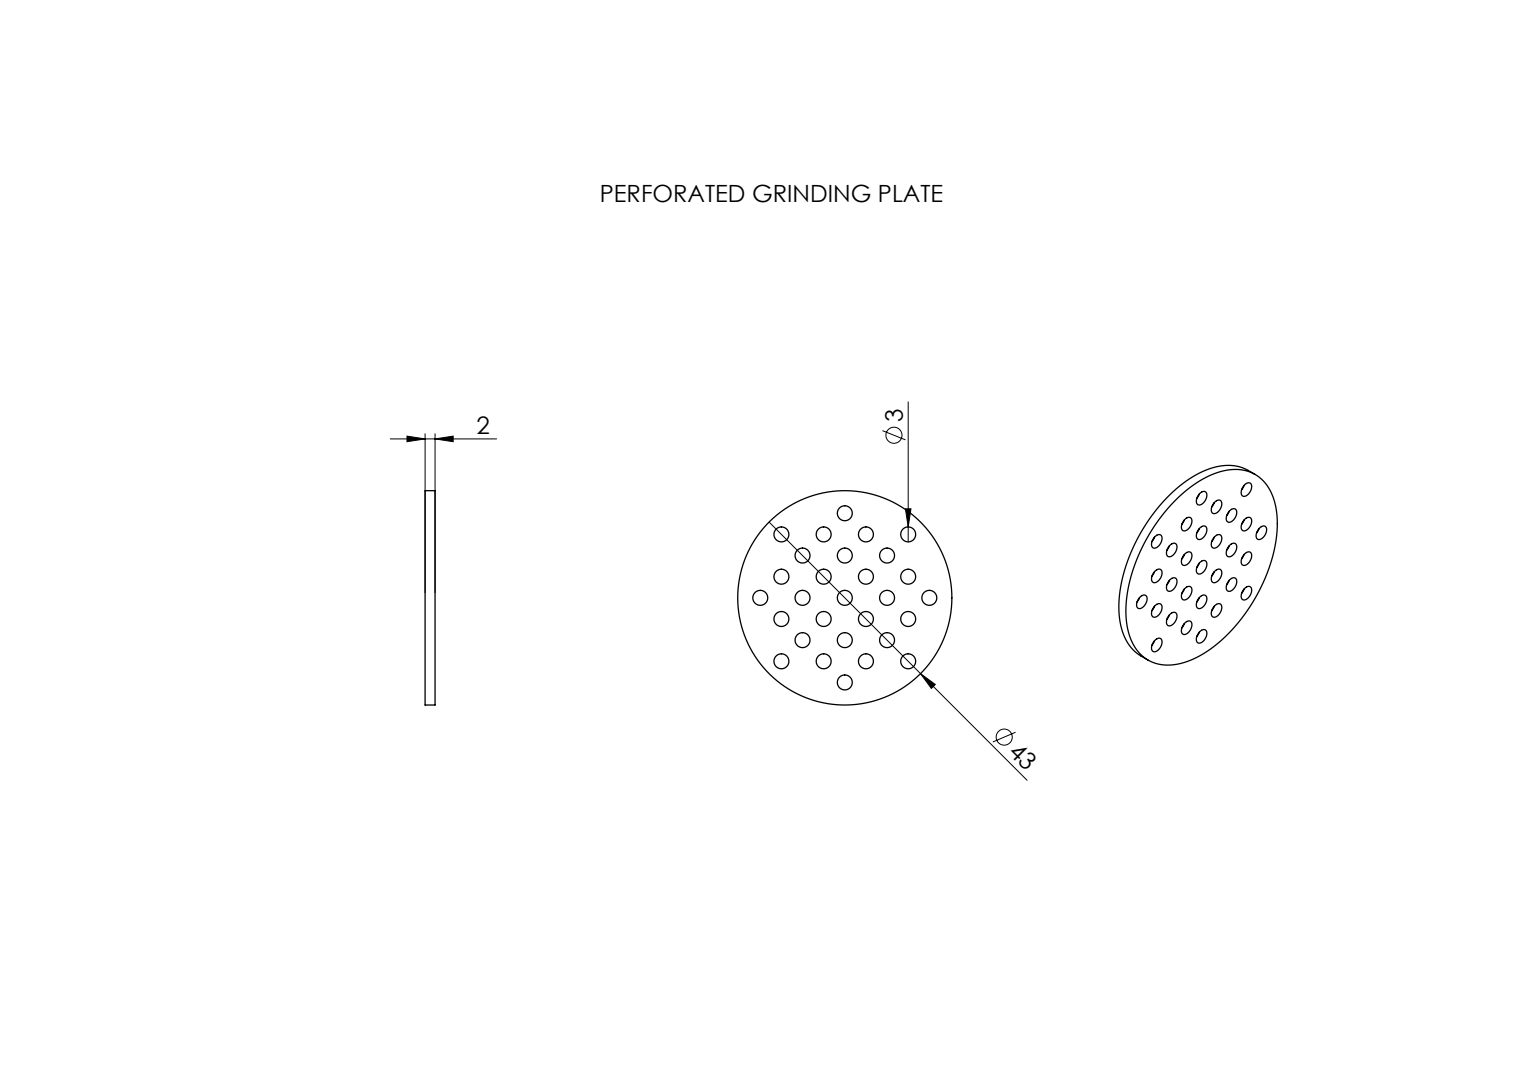
ISO-10303-21;
HEADER;
FILE_DESCRIPTION (('STEP AP214'),
    '1' );
FILE_NAME ('perforated grinding plate.step',
    '2026-10-22T10:02:39',
    ( '' ),
    ( '' ),
    'SwSTEP 2.0',
    'SolidWorks 2026',
    '' );
FILE_SCHEMA (( 'AUTOMOTIVE_DESIGN' ));
ENDSEC;

DATA;
#7=CIRCLE ( 'NONE', #1554, 1.500000000000001332 ) ;
#9=ORIENTED_EDGE ( 'NONE', *, *, #6036, .T. ) ;
#14=AXIS2_PLACEMENT_3D ( 'NONE', #9720, #5068, #10559 ) ;
#19=VERTEX_POINT ( 'NONE', #7735 ) ;
#21=CARTESIAN_POINT ( 'NONE',  ( -78.00000000000001421, 59.24264068711927678, 4.242644059037073312 ) ) ;
#27=DIRECTION ( 'NONE',  ( 0.000000000000000000, 0.000000000000000000, 1.000000000000000000 ) ) ;
#28=CARTESIAN_POINT ( 'NONE',  ( -78.00000000000001421, 50.75735931288069480, -11.22791868944003824 ) ) ;
#29=DIRECTION ( 'NONE',  ( -1.000000000000000000, -0.000000000000000000, -0.000000000000000000 ) ) ;
#34=CARTESIAN_POINT ( 'NONE',  ( -80.00000000000001421, 63.48528137423857487, 8.485284746156350977 ) ) ;
#36=DIRECTION ( 'NONE',  ( 0.000000000000000000, 1.000000000000000000, 0.000000000000000000 ) ) ;
#43=VERTEX_POINT ( 'NONE', #10470 ) ;
#61=ADVANCED_FACE ( 'NONE', ( #1382, #293, #5043, #8690, #5765, #7618, #472, #11246, #4861, #6728, #10360, #351, #7675, #5881, #9524, #9811, #11776, #5272, #7139, #8090, #4373, #7912, #9698, #7079, #1495, #5216, #7192, #9040, #7965, #8982 ), #11541, .F. ) ;
#68=FACE_OUTER_BOUND ( 'NONE', #814, .T. ) ;
#69=VERTEX_POINT ( 'NONE', #11601 ) ;
#72=EDGE_CURVE ( 'NONE', #8769, #5516, #701, .T. ) ;
#79=EDGE_LOOP ( 'NONE', ( #6944, #10404, #6581, #2124 ) ) ;
#88=LINE ( 'NONE', #7135, #10139 ) ;
#89=VERTEX_POINT ( 'NONE', #9752 ) ;
#90=CARTESIAN_POINT ( 'NONE',  ( -78.00000000000002842, 54.99999999999998579, 15.47056612039490986 ) ) ;
#96=VERTEX_POINT ( 'NONE', #6118 ) ;
#102=CARTESIAN_POINT ( 'NONE',  ( -80.00000000000002842, 38.02943725152282184, 3.371917797929946392E-06 ) ) ;
#114=ORIENTED_EDGE ( 'NONE', *, *, #10655, .T. ) ;
#118=CIRCLE ( 'NONE', #8173, 1.500000000000001332 ) ;
#119=CARTESIAN_POINT ( 'NONE',  ( -78.00000000000001421, 50.75735931288069480, -12.72791868944003824 ) ) ;
#128=ORIENTED_EDGE ( 'NONE', *, *, #8290, .T. ) ;
#130=CYLINDRICAL_SURFACE ( 'NONE', #5375, 1.500000000000000000 ) ;
#150=CYLINDRICAL_SURFACE ( 'NONE', #7865, 1.499999999999999556 ) ;
#152=ORIENTED_EDGE ( 'NONE', *, *, #4340, .T. ) ;
#169=CIRCLE ( 'NONE', #3240, 1.500000000000001332 ) ;
#172=AXIS2_PLACEMENT_3D ( 'NONE', #8865, #9866, #7078 ) ;
#183=CYLINDRICAL_SURFACE ( 'NONE', #11845, 1.500000000000000444 ) ;
#195=VECTOR ( 'NONE', #5572, 1000.000000000000000 ) ;
#202=PRESENTATION_STYLE_ASSIGNMENT (( #2843 ) ) ;
#206=EDGE_CURVE ( 'NONE', #6519, #11654, #6983, .T. ) ;
#232=ORIENTED_EDGE ( 'NONE', *, *, #8402, .T. ) ;
#241=VERTEX_POINT ( 'NONE', #2085 ) ;
#244=LINE ( 'NONE', #4871, #4047 ) ;
#245=FACE_BOUND ( 'NONE', #9079, .T. ) ;
#247=DIRECTION ( 'NONE',  ( -1.000000000000000000, -0.000000000000000000, -0.000000000000000000 ) ) ;
#248=DIRECTION ( 'NONE',  ( -1.000000000000000000, -0.000000000000000000, -0.000000000000000000 ) ) ;
#250=CARTESIAN_POINT ( 'NONE',  ( -78.00000000000002842, 42.27207793864211283, -4.242637315201479353 ) ) ;
#252=ORIENTED_EDGE ( 'NONE', *, *, #5075, .F. ) ;
#255=DIRECTION ( 'NONE',  ( -1.000000000000000000, -0.000000000000000000, -0.000000000000000000 ) ) ;
#258=DIRECTION ( 'NONE',  ( 0.000000000000000000, 1.000000000000000000, 0.000000000000000000 ) ) ;
#263=ADVANCED_FACE ( 'NONE', ( #10291 ), #10352, .F. ) ;
#269=CYLINDRICAL_SURFACE ( 'NONE', #2101, 1.499999999999999556 ) ;
#282=DIRECTION ( 'NONE',  ( -1.000000000000000000, -0.000000000000000000, -0.000000000000000000 ) ) ;
#293=FACE_BOUND ( 'NONE', #10060, .T. ) ;
#299=EDGE_CURVE ( 'NONE', #11481, #8007, #11177, .T. ) ;
#302=AXIS2_PLACEMENT_3D ( 'NONE', #9626, #1421, #6826 ) ;
#314=CIRCLE ( 'NONE', #4535, 1.500000000000001332 ) ;
#320=CIRCLE ( 'NONE', #10069, 1.500000000000001332 ) ;
#322=VERTEX_POINT ( 'NONE', #10463 ) ;
#326=EDGE_LOOP ( 'NONE', ( #6442, #4542, #10386, #11390 ) ) ;
#330=CARTESIAN_POINT ( 'NONE',  ( -78.00000000000002842, 42.27207793864211283, -5.742637315201479353 ) ) ;
#332=DIRECTION ( 'NONE',  ( 0.000000000000000000, 0.000000000000000000, 1.000000000000000000 ) ) ;
#334=EDGE_LOOP ( 'NONE', ( #4076, #9464, #9647, #1105 ) ) ;
#341=ORIENTED_EDGE ( 'NONE', *, *, #3274, .F. ) ;
#345=CARTESIAN_POINT ( 'NONE',  ( -78.00000000000001421, 50.75735931288069480, -4.242637315201482906 ) ) ;
#348=EDGE_LOOP ( 'NONE', ( #11086, #2027, #10257, #10094 ) ) ;
#351=FACE_BOUND ( 'NONE', #8937, .T. ) ;
#356=CARTESIAN_POINT ( 'NONE',  ( -80.00000000000002842, 42.27207793864211283, -2.742637315201478909 ) ) ;
#362=AXIS2_PLACEMENT_3D ( 'NONE', #7929, #10661, #6136 ) ;
#369=CARTESIAN_POINT ( 'NONE',  ( -78.00000000000001421, 59.24264068711928388, -12.72791868944003824 ) ) ;
#382=EDGE_CURVE ( 'NONE', #9787, #911, #6720, .T. ) ;
#392=CYLINDRICAL_SURFACE ( 'NONE', #7755, 1.499999999999999556 ) ;
#395=CARTESIAN_POINT ( 'NONE',  ( -78.00000000000002842, 42.27207793864211283, 5.742644059037075088 ) ) ;
#404=ORIENTED_EDGE ( 'NONE', *, *, #2192, .T. ) ;
#411=ORIENTED_EDGE ( 'NONE', *, *, #7065, .F. ) ;
#424=CARTESIAN_POINT ( 'NONE',  ( -78.00000000000001421, 59.24264068711927678, -4.242637315201482906 ) ) ;
#430=VERTEX_POINT ( 'NONE', #4072 ) ;
#441=CARTESIAN_POINT ( 'NONE',  ( -78.00000000000001421, 59.24264068711927678, -4.242637315201482906 ) ) ;
#442=CARTESIAN_POINT ( 'NONE',  ( -78.00000000000001421, 59.24264068711927678, 5.742644059037073312 ) ) ;
#447=EDGE_CURVE ( 'NONE', #3965, #2443, #10013, .T. ) ;
#452=DIRECTION ( 'NONE',  ( -1.000000000000000000, -0.000000000000000000, -0.000000000000000000 ) ) ;
#460=CARTESIAN_POINT ( 'NONE',  ( -78.00000000000000000, 54.99999999999999289, 1.500003371917797201 ) ) ;
#469=ORIENTED_EDGE ( 'NONE', *, *, #6959, .T. ) ;
#471=FACE_OUTER_BOUND ( 'NONE', #3888, .T. ) ;
#472=FACE_BOUND ( 'NONE', #918, .T. ) ;
#479=EDGE_LOOP ( 'NONE', ( #6589, #1548 ) ) ;
#484=ORIENTED_EDGE ( 'NONE', *, *, #797, .F. ) ;
#490=AXIS2_PLACEMENT_3D ( 'NONE', #6892, #11533, #10461 ) ;
#491=EDGE_LOOP ( 'NONE', ( #6034, #9162, #10252, #4142 ) ) ;
#506=AXIS2_PLACEMENT_3D ( 'NONE', #833, #7216, #2766 ) ;
#512=ADVANCED_FACE ( 'NONE', ( #9745 ), #11473, .F. ) ;
#513=CYLINDRICAL_SURFACE ( 'NONE', #1318, 1.499999999999999556 ) ;
#517=AXIS2_PLACEMENT_3D ( 'NONE', #9788, #1581, #2488 ) ;
#518=VERTEX_POINT ( 'NONE', #5210 ) ;
#528=FACE_BOUND ( 'NONE', #6654, .T. ) ;
#537=DIRECTION ( 'NONE',  ( -1.000000000000000000, -0.000000000000000000, -0.000000000000000000 ) ) ;
#540=CYLINDRICAL_SURFACE ( 'NONE', #2889, 1.499999999999999556 ) ;
#548=DIRECTION ( 'NONE',  ( -1.000000000000000000, -0.000000000000000000, -0.000000000000000000 ) ) ;
#554=AXIS2_PLACEMENT_3D ( 'NONE', #4747, #2103, #5776 ) ;
#560=DIRECTION ( 'NONE',  ( -1.000000000000000000, -0.000000000000000000, -0.000000000000000000 ) ) ;
#571=ORIENTED_EDGE ( 'NONE', *, *, #3449, .F. ) ;
#572=AXIS2_PLACEMENT_3D ( 'NONE', #3732, #4757, #2835 ) ;
#575=ORIENTED_EDGE ( 'NONE', *, *, #6777, .T. ) ;
#581=DIRECTION ( 'NONE',  ( -1.000000000000000000, -0.000000000000000000, -0.000000000000000000 ) ) ;
#583=EDGE_LOOP ( 'NONE', ( #10142, #10451 ) ) ;
#587=EDGE_CURVE ( 'NONE', #96, #430, #9252, .T. ) ;
#590=VECTOR ( 'NONE', #3641, 1000.000000000000000 ) ;
#591=ORIENTED_EDGE ( 'NONE', *, *, #3891, .F. ) ;
#600=CYLINDRICAL_SURFACE ( 'NONE', #4784, 1.499999999999999556 ) ;
#615=DIRECTION ( 'NONE',  ( -1.000000000000000000, -0.000000000000000000, -0.000000000000000000 ) ) ;
#622=ORIENTED_EDGE ( 'NONE', *, *, #9614, .F. ) ;
#626=ORIENTED_EDGE ( 'NONE', *, *, #8896, .F. ) ;
#631=ORIENTED_EDGE ( 'NONE', *, *, #4619, .T. ) ;
#635=EDGE_LOOP ( 'NONE', ( #794, #9910 ) ) ;
#640=CARTESIAN_POINT ( 'NONE',  ( -78.00000000000002842, 46.51471862576140381, 1.500003371917798756 ) ) ;
#642=VERTEX_POINT ( 'NONE', #2683 ) ;
#650=CARTESIAN_POINT ( 'NONE',  ( -78.00000000000000000, 54.99999999999999289, 3.371917797062584654E-06 ) ) ;
#656=VERTEX_POINT ( 'NONE', #1719 ) ;
#660=ADVANCED_FACE ( 'NONE', ( #2854 ), #866, .F. ) ;
#666=ORIENTED_EDGE ( 'NONE', *, *, #2138, .F. ) ;
#669=CARTESIAN_POINT ( 'NONE',  ( -78.00000000000001421, 63.48528137423857487, 3.371917795327861178E-06 ) ) ;
#676=FACE_OUTER_BOUND ( 'NONE', #7285, .T. ) ;
#687=AXIS2_PLACEMENT_3D ( 'NONE', #9704, #7974, #8697 ) ;
#688=CARTESIAN_POINT ( 'NONE',  ( -78.00000000000001421, 71.97056274847716395, 3.371917795327861178E-06 ) ) ;
#700=DIRECTION ( 'NONE',  ( -1.000000000000000000, -0.000000000000000000, -0.000000000000000000 ) ) ;
#701=LINE ( 'NONE', #8025, #1937 ) ;
#704=ORIENTED_EDGE ( 'NONE', *, *, #10995, .F. ) ;
#709=DIRECTION ( 'NONE',  ( -1.000000000000000000, -0.000000000000000000, -0.000000000000000000 ) ) ;
#715=EDGE_LOOP ( 'NONE', ( #11097, #2302, #10666, #3336 ) ) ;
#721=DIRECTION ( 'NONE',  ( -1.000000000000000000, -0.000000000000000000, -0.000000000000000000 ) ) ;
#723=VERTEX_POINT ( 'NONE', #1773 ) ;
#727=DIRECTION ( 'NONE',  ( -1.000000000000000000, -0.000000000000000000, -0.000000000000000000 ) ) ;
#731=EDGE_LOOP ( 'NONE', ( #2625, #3077 ) ) ;
#749=ORIENTED_EDGE ( 'NONE', *, *, #5956, .F. ) ;
#753=DIRECTION ( 'NONE',  ( -1.000000000000000000, -0.000000000000000000, -0.000000000000000000 ) ) ;
#754=DIRECTION ( 'NONE',  ( -1.000000000000000000, -0.000000000000000000, -0.000000000000000000 ) ) ;
#758=DIRECTION ( 'NONE',  ( 1.000000000000000000, 0.000000000000000000, 0.000000000000000000 ) ) ;
#762=CARTESIAN_POINT ( 'NONE',  ( -78.00000000000002842, 50.75735931288069480, 2.742644059037076865 ) ) ;
#770=ORIENTED_EDGE ( 'NONE', *, *, #9291, .F. ) ;
#771=FACE_OUTER_BOUND ( 'NONE', #5097, .T. ) ;
#773=ORIENTED_EDGE ( 'NONE', *, *, #9797, .T. ) ;
#780=VECTOR ( 'NONE', #11369, 1000.000000000000000 ) ;
#781=CARTESIAN_POINT ( 'NONE',  ( -80.00000000000002842, 42.27207793864211283, 4.242644059037075976 ) ) ;
#782=ORIENTED_EDGE ( 'NONE', *, *, #7210, .T. ) ;
#785=ADVANCED_FACE ( 'NONE', ( #1357 ), #392, .F. ) ;
#794=ORIENTED_EDGE ( 'NONE', *, *, #4701, .F. ) ;
#797=EDGE_CURVE ( 'NONE', #10685, #2528, #2250, .T. ) ;
#798=EDGE_CURVE ( 'NONE', #1970, #8495, #11569, .T. ) ;
#803=ADVANCED_FACE ( 'NONE', ( #4958 ), #1174, .F. ) ;
#804=EDGE_CURVE ( 'NONE', #19, #11526, #11182, .T. ) ;
#805=DIRECTION ( 'NONE',  ( -1.000000000000000000, -0.000000000000000000, -0.000000000000000000 ) ) ;
#814=EDGE_LOOP ( 'NONE', ( #11632, #7183, #5168, #5466 ) ) ;
#828=ORIENTED_EDGE ( 'NONE', *, *, #4635, .T. ) ;
#833=CARTESIAN_POINT ( 'NONE',  ( -78.00000000000001421, 42.27207793864211283, -12.72791868944003824 ) ) ;
#839=EDGE_CURVE ( 'NONE', #5641, #4778, #6767, .T. ) ;
#849=VERTEX_POINT ( 'NONE', #7717 ) ;
#857=SHAPE_REPRESENTATION_RELATIONSHIP ( 'NONE' , 'NONE' ,  #3715, #1113 ) ;
#861=CIRCLE ( 'NONE', #9487, 1.500000000000001332 ) ;
#862=ORIENTED_EDGE ( 'NONE', *, *, #587, .F. ) ;
#866=CYLINDRICAL_SURFACE ( 'NONE', #6599, 1.499999999999999556 ) ;
#874=VECTOR ( 'NONE', #8482, 1000.000000000000000 ) ;
#877=CYLINDRICAL_SURFACE ( 'NONE', #4723, 1.500000000000000000 ) ;
#880=CARTESIAN_POINT ( 'NONE',  ( -80.00000000000001421, 67.72792206135787296, -11.22791868944004534 ) ) ;
#881=DIRECTION ( 'NONE',  ( -1.000000000000000000, -0.000000000000000000, -0.000000000000000000 ) ) ;
#893=FACE_OUTER_BOUND ( 'NONE', #5900, .T. ) ;
#895=AXIS2_PLACEMENT_3D ( 'NONE', #11702, #4576, #8117 ) ;
#908=ORIENTED_EDGE ( 'NONE', *, *, #2554, .T. ) ;
#911=VERTEX_POINT ( 'NONE', #7767 ) ;
#916=( NAMED_UNIT ( * ) SI_UNIT ( $, .STERADIAN. ) SOLID_ANGLE_UNIT ( ) );
#917=AXIS2_PLACEMENT_3D ( 'NONE', #6828, #10454, #10804 ) ;
#918=EDGE_LOOP ( 'NONE', ( #7409, #3396 ) ) ;
#920=FACE_OUTER_BOUND ( 'NONE', #10715, .T. ) ;
#929=DIRECTION ( 'NONE',  ( 0.000000000000000000, 0.000000000000000000, 1.000000000000000000 ) ) ;
#930=CARTESIAN_POINT ( 'NONE',  ( -78.00000000000001421, 63.48528137423857487, 6.985284746156351865 ) ) ;
#932=VERTEX_POINT ( 'NONE', #10728 ) ;
#938=AXIS2_PLACEMENT_3D ( 'NONE', #11200, #1023, #6006 ) ;
#950=ORIENTED_EDGE ( 'NONE', *, *, #804, .T. ) ;
#956=EDGE_CURVE ( 'NONE', #9492, #656, #6378, .T. ) ;
#957=ADVANCED_FACE ( 'NONE', ( #1749 ), #7221, .F. ) ;
#959=EDGE_LOOP ( 'NONE', ( #4734, #11437 ) ) ;
#960=EDGE_CURVE ( 'NONE', #2363, #8766, #6620, .T. ) ;
#965=AXIS2_PLACEMENT_3D ( 'NONE', #5635, #6779, #4790 ) ;
#968=DIRECTION ( 'NONE',  ( -1.000000000000000000, -0.000000000000000000, -0.000000000000000000 ) ) ;
#974=ORIENTED_EDGE ( 'NONE', *, *, #11026, .T. ) ;
#979=ORIENTED_EDGE ( 'NONE', *, *, #1682, .T. ) ;
#983=( NAMED_UNIT ( * ) SI_UNIT ( $, .STERADIAN. ) SOLID_ANGLE_UNIT ( ) );
#994=DIRECTION ( 'NONE',  ( -1.000000000000000000, -0.000000000000000000, -0.000000000000000000 ) ) ;
#1003=ORIENTED_EDGE ( 'NONE', *, *, #10279, .T. ) ;
#1023=DIRECTION ( 'NONE',  ( -1.000000000000000000, -0.000000000000000000, -0.000000000000000000 ) ) ;
#1030=EDGE_CURVE ( 'NONE', #9436, #2186, #169, .T. ) ;
#1031=DIRECTION ( 'NONE',  ( -1.000000000000000000, -0.000000000000000000, -0.000000000000000000 ) ) ;
#1033=VERTEX_POINT ( 'NONE', #6491 ) ;
#1046=EDGE_LOOP ( 'NONE', ( #7442, #8022 ) ) ;
#1061=CARTESIAN_POINT ( 'NONE',  ( -78.00000000000001421, 67.72792206135787296, 4.242644059037073312 ) ) ;
#1065=DIRECTION ( 'NONE',  ( 0.000000000000000000, 1.000000000000000000, 0.000000000000000000 ) ) ;
#1068=ORIENTED_EDGE ( 'NONE', *, *, #6473, .F. ) ;
#1070=ORIENTED_EDGE ( 'NONE', *, *, #9812, .T. ) ;
#1075=CARTESIAN_POINT ( 'NONE',  ( -78.00000000000001421, 50.75735931288069480, -12.72791868944003824 ) ) ;
#1076=EDGE_CURVE ( 'NONE', #3494, #10599, #10880, .T. ) ;
#1085=FACE_BOUND ( 'NONE', #2514, .T. ) ;
#1088=CIRCLE ( 'NONE', #7236, 1.500000000000001332 ) ;
#1091=CYLINDRICAL_SURFACE ( 'NONE', #6278, 1.500000000000000000 ) ;
#1093=LINE ( 'NONE', #10317, #4033 ) ;
#1097=AXIS2_PLACEMENT_3D ( 'NONE', #8579, #2100, #4867 ) ;
#1102=CARTESIAN_POINT ( 'NONE',  ( -78.00000000000002842, 38.02943725152282184, 3.371917797929946392E-06 ) ) ;
#1105=ORIENTED_EDGE ( 'NONE', *, *, #11853, .T. ) ;
#1109=DIRECTION ( 'NONE',  ( -1.000000000000000000, -0.000000000000000000, -0.000000000000000000 ) ) ;
#1113=ADVANCED_BREP_SHAPE_REPRESENTATION ( '', ( #8587, #4738 ), #2442 ) ;
#1118=DIRECTION ( 'NONE',  ( -1.000000000000000000, -0.000000000000000000, -0.000000000000000000 ) ) ;
#1120=AXIS2_PLACEMENT_3D ( 'NONE', #1648, #2557, #3689 ) ;
#1128=ORIENTED_EDGE ( 'NONE', *, *, #8880, .T. ) ;
#1137=AXIS2_PLACEMENT_3D ( 'NONE', #1291, #3153, #8722 ) ;
#1142=FACE_BOUND ( 'NONE', #2463, .T. ) ;
#1149=CYLINDRICAL_SURFACE ( 'NONE', #8557, 1.499999999999999556 ) ;
#1152=EDGE_CURVE ( 'NONE', #8509, #1264, #2669, .T. ) ;
#1158=CARTESIAN_POINT ( 'NONE',  ( -80.00000000000002842, 59.24264068711927678, 12.72792543327563131 ) ) ;
#1162=ORIENTED_EDGE ( 'NONE', *, *, #1324, .F. ) ;
#1172=AXIS2_PLACEMENT_3D ( 'NONE', #5050, #537, #4201 ) ;
#1174=CYLINDRICAL_SURFACE ( 'NONE', #4688, 1.499999999999999556 ) ;
#1180=DIRECTION ( 'NONE',  ( -1.000000000000000000, -0.000000000000000000, -0.000000000000000000 ) ) ;
#1181=EDGE_CURVE ( 'NONE', #10867, #4978, #10110, .T. ) ;
#1183=AXIS2_PLACEMENT_3D ( 'NONE', #6561, #7279, #2718 ) ;
#1192=DIRECTION ( 'NONE',  ( -1.000000000000000000, -0.000000000000000000, -0.000000000000000000 ) ) ;
#1202=CARTESIAN_POINT ( 'NONE',  ( -78.00000000000002842, 50.75735931288069480, 4.242644059037076865 ) ) ;
#1203=ORIENTED_EDGE ( 'NONE', *, *, #2554, .F. ) ;
#1214=EDGE_LOOP ( 'NONE', ( #11185, #4171, #3721, #9359 ) ) ;
#1229=CARTESIAN_POINT ( 'NONE',  ( -78.00000000000001421, 59.24264068711927678, -2.742637315201482462 ) ) ;
#1236=CARTESIAN_POINT ( 'NONE',  ( -80.00000000000001421, 59.24264068711927678, -4.242637315201482906 ) ) ;
#1239=ORIENTED_EDGE ( 'NONE', *, *, #9815, .F. ) ;
#1243=DIRECTION ( 'NONE',  ( 0.000000000000000000, 0.000000000000000000, 1.000000000000000000 ) ) ;
#1244=DIRECTION ( 'NONE',  ( -1.000000000000000000, -0.000000000000000000, -0.000000000000000000 ) ) ;
#1250=ORIENTED_EDGE ( 'NONE', *, *, #4162, .T. ) ;
#1251=DIRECTION ( 'NONE',  ( 0.000000000000000000, 1.000000000000000000, 0.000000000000000000 ) ) ;
#1257=ORIENTED_EDGE ( 'NONE', *, *, #6099, .T. ) ;
#1262=VECTOR ( 'NONE', #11203, 1000.000000000000000 ) ;
#1264=VERTEX_POINT ( 'NONE', #11719 ) ;
#1269=LINE ( 'NONE', #10251, #1262 ) ;
#1277=DIRECTION ( 'NONE',  ( -1.000000000000000000, -0.000000000000000000, -0.000000000000000000 ) ) ;
#1278=DIRECTION ( 'NONE',  ( 0.000000000000000000, 1.000000000000000000, 0.000000000000000000 ) ) ;
#1285=DIRECTION ( 'NONE',  ( -1.000000000000000000, -0.000000000000000000, -0.000000000000000000 ) ) ;
#1291=CARTESIAN_POINT ( 'NONE',  ( -78.00000000000001421, 63.48528137423857487, 3.371917795327861178E-06 ) ) ;
#1293=VECTOR ( 'NONE', #9725, 1000.000000000000000 ) ;
#1294=EDGE_CURVE ( 'NONE', #322, #6131, #3340, .T. ) ;
#1301=CARTESIAN_POINT ( 'NONE',  ( -80.00000000000001421, 42.27207793864211283, -12.72791868944003824 ) ) ;
#1307=DIRECTION ( 'NONE',  ( 0.000000000000000000, 1.000000000000000000, 0.000000000000000000 ) ) ;
#1312=VERTEX_POINT ( 'NONE', #640 ) ;
#1318=AXIS2_PLACEMENT_3D ( 'NONE', #8730, #6167, #10625 ) ;
#1320=DIRECTION ( 'NONE',  ( 0.000000000000000000, 1.000000000000000000, 0.000000000000000000 ) ) ;
#1324=EDGE_CURVE ( 'NONE', #430, #96, #1885, .T. ) ;
#1328=AXIS2_PLACEMENT_3D ( 'NONE', #3473, #2386, #8089 ) ;
#1330=ORIENTED_EDGE ( 'NONE', *, *, #4547, .T. ) ;
#1332=EDGE_CURVE ( 'NONE', #8286, #8080, #3287, .T. ) ;
#1334=CARTESIAN_POINT ( 'NONE',  ( -78.00000000000001421, 63.48528137423857487, -9.985278002320759683 ) ) ;
#1345=LINE ( 'NONE', #5009, #6940 ) ;
#1357=FACE_OUTER_BOUND ( 'NONE', #3937, .T. ) ;
#1358=AXIS2_PLACEMENT_3D ( 'NONE', #10716, #3305, #9829 ) ;
#1359=CARTESIAN_POINT ( 'NONE',  ( -78.00000000000002842, 46.51471862576140381, 1.500003371917798756 ) ) ;
#1366=AXIS2_PLACEMENT_3D ( 'NONE', #3867, #255, #11093 ) ;
#1380=FACE_BOUND ( 'NONE', #6482, .T. ) ;
#1381=AXIS2_PLACEMENT_3D ( 'NONE', #11447, #7816, #6146 ) ;
#1382=FACE_BOUND ( 'NONE', #8062, .T. ) ;
#1383=DIRECTION ( 'NONE',  ( 1.000000000000000000, 0.000000000000000000, 0.000000000000000000 ) ) ;
#1389=CARTESIAN_POINT ( 'NONE',  ( -78.00000000000002842, 50.75735931288069480, 5.742644059037076865 ) ) ;
#1393=EDGE_LOOP ( 'NONE', ( #5631, #3625 ) ) ;
#1396=DIRECTION ( 'NONE',  ( 0.000000000000000000, 1.000000000000000000, 0.000000000000000000 ) ) ;
#1400=ORIENTED_EDGE ( 'NONE', *, *, #2192, .F. ) ;
#1403=CARTESIAN_POINT ( 'NONE',  ( -78.00000000000002842, 59.24264068711927678, 11.22792543327563131 ) ) ;
#1408=EDGE_CURVE ( 'NONE', #932, #11654, #10812, .T. ) ;
#1417=CARTESIAN_POINT ( 'NONE',  ( -78.00000000000002842, 46.51471862576140381, 8.485284746156354529 ) ) ;
#1421=DIRECTION ( 'NONE',  ( -1.000000000000000000, -0.000000000000000000, -0.000000000000000000 ) ) ;
#1423=LINE ( 'NONE', #460, #11019 ) ;
#1441=AXIS2_PLACEMENT_3D ( 'NONE', #1417, #1628, #5294 ) ;
#1443=CARTESIAN_POINT ( 'NONE',  ( -80.00000000000002842, 42.27207793864211283, 14.22792543327562775 ) ) ;
#1448=ORIENTED_EDGE ( 'NONE', *, *, #2574, .T. ) ;
#1460=EDGE_CURVE ( 'NONE', #2849, #8906, #2855, .T. ) ;
#1468=CARTESIAN_POINT ( 'NONE',  ( -78.00000000000002842, 50.75735931288069480, 11.22792543327563131 ) ) ;
#1474=AXIS2_PLACEMENT_3D ( 'NONE', #5522, #7565, #3064 ) ;
#1475=AXIS2_PLACEMENT_3D ( 'NONE', #345, #4914, #2086 ) ;
#1484=ORIENTED_EDGE ( 'NONE', *, *, #3072, .T. ) ;
#1492=VERTEX_POINT ( 'NONE', #6350 ) ;
#1494=CARTESIAN_POINT ( 'NONE',  ( -78.00000000000000000, 55.00000000000000000, 0.000000000000000000 ) ) ;
#1495=FACE_BOUND ( 'NONE', #2402, .T. ) ;
#1513=ORIENTED_EDGE ( 'NONE', *, *, #11196, .T. ) ;
#1516=DIRECTION ( 'NONE',  ( -1.000000000000000000, -0.000000000000000000, -0.000000000000000000 ) ) ;
#1525=EDGE_CURVE ( 'NONE', #1807, #3299, #8194, .T. ) ;
#1536=CARTESIAN_POINT ( 'NONE',  ( -78.00000000000002842, 54.99999999999998579, 8.485284746156354529 ) ) ;
#1539=EDGE_LOOP ( 'NONE', ( #5443, #8996, #8262, #9 ) ) ;
#1542=FACE_OUTER_BOUND ( 'NONE', #491, .T. ) ;
#1546=AXIS2_PLACEMENT_3D ( 'NONE', #7939, #968, #5419 ) ;
#1548=ORIENTED_EDGE ( 'NONE', *, *, #5066, .F. ) ;
#1553=ORIENTED_EDGE ( 'NONE', *, *, #2286, .F. ) ;
#1554=AXIS2_PLACEMENT_3D ( 'NONE', #2158, #9281, #11250 ) ;
#1557=EDGE_CURVE ( 'NONE', #2610, #4492, #10091, .T. ) ;
#1561=AXIS2_PLACEMENT_3D ( 'NONE', #9701, #1608, #6009 ) ;
#1564=DIRECTION ( 'NONE',  ( -1.000000000000000000, -0.000000000000000000, -0.000000000000000000 ) ) ;
#1581=DIRECTION ( 'NONE',  ( -1.000000000000000000, -0.000000000000000000, -0.000000000000000000 ) ) ;
#1590=ORIENTED_EDGE ( 'NONE', *, *, #299, .T. ) ;
#1592=ADVANCED_FACE ( 'NONE', ( #7420 ), #9088, .F. ) ;
#1599=CARTESIAN_POINT ( 'NONE',  ( -78.00000000000001421, 71.97056274847716395, -1.499996628082204797 ) ) ;
#1602=ORIENTED_EDGE ( 'NONE', *, *, #3934, .T. ) ;
#1608=DIRECTION ( 'NONE',  ( -1.000000000000000000, -0.000000000000000000, -0.000000000000000000 ) ) ;
#1611=DIRECTION ( 'NONE',  ( 0.000000000000000000, 0.000000000000000000, 1.000000000000000000 ) ) ;
#1615=DIRECTION ( 'NONE',  ( 0.000000000000000000, 0.000000000000000000, 1.000000000000000000 ) ) ;
#1616=ORIENTED_EDGE ( 'NONE', *, *, #839, .T. ) ;
#1617=DIRECTION ( 'NONE',  ( -1.000000000000000000, -0.000000000000000000, -0.000000000000000000 ) ) ;
#1618=VERTEX_POINT ( 'NONE', #10216 ) ;
#1622=DIRECTION ( 'NONE',  ( 0.000000000000000000, 1.000000000000000000, 0.000000000000000000 ) ) ;
#1628=DIRECTION ( 'NONE',  ( -1.000000000000000000, -0.000000000000000000, -0.000000000000000000 ) ) ;
#1648=CARTESIAN_POINT ( 'NONE',  ( -80.00000000000001421, 63.48528137423857487, 3.371917795327861178E-06 ) ) ;
#1651=EDGE_LOOP ( 'NONE', ( #7480, #11260, #3913, #11469 ) ) ;
#1661=DIRECTION ( 'NONE',  ( 1.000000000000000000, 0.000000000000000000, 0.000000000000000000 ) ) ;
#1666=AXIS2_PLACEMENT_3D ( 'NONE', #2364, #560, #2303 ) ;
#1670=LINE ( 'NONE', #11732, #5906 ) ;
#1674=( GEOMETRIC_REPRESENTATION_CONTEXT ( 3 ) GLOBAL_UNCERTAINTY_ASSIGNED_CONTEXT ( ( #5920 ) ) GLOBAL_UNIT_ASSIGNED_CONTEXT ( ( #6512, #6394, #916 ) ) REPRESENTATION_CONTEXT ( 'NONE', 'WORKASPACE' ) );
#1682=EDGE_CURVE ( 'NONE', #518, #6038, #6128, .T. ) ;
#1685=EDGE_CURVE ( 'NONE', #10685, #1618, #2483, .T. ) ;
#1687=CARTESIAN_POINT ( 'NONE',  ( -80.00000000000002842, 42.27207793864211283, -5.742637315201479353 ) ) ;
#1692=EDGE_CURVE ( 'NONE', #7395, #5447, #9503, .T. ) ;
#1698=ADVANCED_FACE ( 'NONE', ( #7540 ), #3997, .F. ) ;
#1699=ORIENTED_EDGE ( 'NONE', *, *, #5066, .T. ) ;
#1702=EDGE_LOOP ( 'NONE', ( #4407, #4118 ) ) ;
#1706=VERTEX_POINT ( 'NONE', #5807 ) ;
#1710=DIRECTION ( 'NONE',  ( -1.000000000000000000, -0.000000000000000000, -0.000000000000000000 ) ) ;
#1714=AXIS2_PLACEMENT_3D ( 'NONE', #6464, #754, #11720 ) ;
#1719=CARTESIAN_POINT ( 'NONE',  ( -80.00000000000002842, 42.27207793864211283, 2.742644059037075976 ) ) ;
#1722=ORIENTED_EDGE ( 'NONE', *, *, #1915, .T. ) ;
#1724=CARTESIAN_POINT ( 'NONE',  ( -78.00000000000001421, 59.24264068711928388, -12.72791868944003824 ) ) ;
#1725=DIRECTION ( 'NONE',  ( 0.000000000000000000, 0.000000000000000000, -1.000000000000000000 ) ) ;
#1731=EDGE_CURVE ( 'NONE', #1492, #6194, #6507, .T. ) ;
#1737=ORIENTED_EDGE ( 'NONE', *, *, #1076, .F. ) ;
#1740=ORIENTED_EDGE ( 'NONE', *, *, #6906, .F. ) ;
#1749=FACE_OUTER_BOUND ( 'NONE', #5704, .T. ) ;
#1751=DIRECTION ( 'NONE',  ( -1.000000000000000000, -0.000000000000000000, -0.000000000000000000 ) ) ;
#1757=DIRECTION ( 'NONE',  ( -1.000000000000000000, -0.000000000000000000, -0.000000000000000000 ) ) ;
#1758=ORIENTED_EDGE ( 'NONE', *, *, #11718, .F. ) ;
#1762=CARTESIAN_POINT ( 'NONE',  ( -80.00000000000001421, 67.72792206135787296, 5.742644059037073312 ) ) ;
#1765=EDGE_CURVE ( 'NONE', #1312, #11779, #8616, .T. ) ;
#1767=ORIENTED_EDGE ( 'NONE', *, *, #299, .F. ) ;
#1768=CYLINDRICAL_SURFACE ( 'NONE', #9732, 1.500000000000001332 ) ;
#1770=VERTEX_POINT ( 'NONE', #2977 ) ;
#1773=CARTESIAN_POINT ( 'NONE',  ( -80.00000000000001421, 54.99999999999999289, -18.47055937655931501 ) ) ;
#1792=ORIENTED_EDGE ( 'NONE', *, *, #10967, .T. ) ;
#1798=VERTEX_POINT ( 'NONE', #6880 ) ;
#1807=VERTEX_POINT ( 'NONE', #395 ) ;
#1816=FILL_AREA_STYLE_COLOUR ( '', #8758 ) ;
#1818=DIRECTION ( 'NONE',  ( 0.000000000000000000, 0.000000000000000000, 1.000000000000000000 ) ) ;
#1826=( NAMED_UNIT ( * ) SI_UNIT ( $, .STERADIAN. ) SOLID_ANGLE_UNIT ( ) );
#1828=VECTOR ( 'NONE', #11433, 1000.000000000000000 ) ;
#1830=DIRECTION ( 'NONE',  ( 0.000000000000000000, 0.000000000000000000, 1.000000000000000000 ) ) ;
#1831=VERTEX_POINT ( 'NONE', #3653 ) ;
#1839=AXIS2_PLACEMENT_3D ( 'NONE', #10418, #6010, #4133 ) ;
#1841=ORIENTED_EDGE ( 'NONE', *, *, #10879, .T. ) ;
#1850=VERTEX_POINT ( 'NONE', #4609 ) ;
#1857=CIRCLE ( 'NONE', #7994, 1.500000000000001332 ) ;
#1868=EDGE_LOOP ( 'NONE', ( #979, #6937 ) ) ;
#1871=EDGE_CURVE ( 'NONE', #6614, #8495, #10170, .T. ) ;
#1878=CARTESIAN_POINT ( 'NONE',  ( -80.00000000000002842, 42.27207793864211283, 4.242644059037075976 ) ) ;
#1885=CIRCLE ( 'NONE', #3057, 1.500000000000001332 ) ;
#1889=CIRCLE ( 'NONE', #6318, 21.50000000000000000 ) ;
#1895=PRODUCT_DEFINITION ( 'UNKNOWN', '', #7575, #7866 ) ;
#1914=ADVANCED_FACE ( 'NONE', ( #7318 ), #10945, .F. ) ;
#1915=EDGE_CURVE ( 'NONE', #2443, #3965, #6530, .T. ) ;
#1918=CIRCLE ( 'NONE', #3844, 1.500000000000001332 ) ;
#1919=FACE_OUTER_BOUND ( 'NONE', #5973, .T. ) ;
#1920=ORIENTED_EDGE ( 'NONE', *, *, #5579, .T. ) ;
#1930=DIRECTION ( 'NONE',  ( -1.000000000000000000, -0.000000000000000000, -0.000000000000000000 ) ) ;
#1937=VECTOR ( 'NONE', #3474, 1000.000000000000000 ) ;
#1954=DIRECTION ( 'NONE',  ( -1.000000000000000000, -0.000000000000000000, -0.000000000000000000 ) ) ;
#1964=DIRECTION ( 'NONE',  ( -1.000000000000000000, -0.000000000000000000, -0.000000000000000000 ) ) ;
#1970=VERTEX_POINT ( 'NONE', #7370 ) ;
#1977=CARTESIAN_POINT ( 'NONE',  ( -78.00000000000001421, 54.99999999999999289, -16.97055937655931501 ) ) ;
#1984=FACE_BOUND ( 'NONE', #10175, .T. ) ;
#2011=ORIENTED_EDGE ( 'NONE', *, *, #10767, .T. ) ;
#2023=DIRECTION ( 'NONE',  ( -1.000000000000000000, -0.000000000000000000, -0.000000000000000000 ) ) ;
#2027=ORIENTED_EDGE ( 'NONE', *, *, #9346, .T. ) ;
#2032=AXIS2_PLACEMENT_3D ( 'NONE', #11264, #3076, #6746 ) ;
#2038=PRODUCT ( 'perforated grinding plate', 'perforated grinding plate', '', ( #6496 ) ) ;
#2042=CIRCLE ( 'NONE', #4539, 1.500000000000001332 ) ;
#2044=FACE_BOUND ( 'NONE', #8189, .T. ) ;
#2056=CARTESIAN_POINT ( 'NONE',  ( -78.00000000000002842, 46.51471862576140381, 6.985284746156355418 ) ) ;
#2059=AXIS2_PLACEMENT_3D ( 'NONE', #9874, #2754, #10709 ) ;
#2072=CARTESIAN_POINT ( 'NONE',  ( -78.00000000000002842, 59.24264068711927678, 14.22792543327563131 ) ) ;
#2085=CARTESIAN_POINT ( 'NONE',  ( -80.00000000000001421, 63.48528137423857487, -6.985278002320760571 ) ) ;
#2086=DIRECTION ( 'NONE',  ( 0.000000000000000000, 1.000000000000000000, 0.000000000000000000 ) ) ;
#2094=AXIS2_PLACEMENT_3D ( 'NONE', #3231, #8918, #2569 ) ;
#2098=APPLICATION_CONTEXT ( 'automotive_design' ) ;
#2099=DIRECTION ( 'NONE',  ( -1.000000000000000000, -0.000000000000000000, -0.000000000000000000 ) ) ;
#2100=DIRECTION ( 'NONE',  ( -1.000000000000000000, -0.000000000000000000, -0.000000000000000000 ) ) ;
#2101=AXIS2_PLACEMENT_3D ( 'NONE', #9621, #10568, #7716 ) ;
#2102=EDGE_LOOP ( 'NONE', ( #11444, #8277 ) ) ;
#2103=DIRECTION ( 'NONE',  ( -1.000000000000000000, -0.000000000000000000, -0.000000000000000000 ) ) ;
#2112=VECTOR ( 'NONE', #8051, 1000.000000000000000 ) ;
#2113=DIRECTION ( 'NONE',  ( -1.000000000000000000, -0.000000000000000000, -0.000000000000000000 ) ) ;
#2114=ORIENTED_EDGE ( 'NONE', *, *, #2937, .T. ) ;
#2120=CIRCLE ( 'NONE', #1358, 1.500000000000001332 ) ;
#2124=ORIENTED_EDGE ( 'NONE', *, *, #6188, .T. ) ;
#2133=AXIS2_PLACEMENT_3D ( 'NONE', #5955, #5108, #10649 ) ;
#2138=EDGE_CURVE ( 'NONE', #4578, #911, #4217, .T. ) ;
#2143=CYLINDRICAL_SURFACE ( 'NONE', #4623, 1.500000000000000000 ) ;
#2148=CARTESIAN_POINT ( 'NONE',  ( -78.00000000000001421, 50.75735931288069480, -2.742637315201482462 ) ) ;
#2149=CARTESIAN_POINT ( 'NONE',  ( -78.00000000000002842, 50.75735931288069480, 14.22792543327563131 ) ) ;
#2153=ORIENTED_EDGE ( 'NONE', *, *, #1324, .T. ) ;
#2155=ORIENTED_EDGE ( 'NONE', *, *, #1692, .F. ) ;
#2158=CARTESIAN_POINT ( 'NONE',  ( -78.00000000000001421, 63.48528137423857487, 8.485284746156350977 ) ) ;
#2160=DIRECTION ( 'NONE',  ( -1.000000000000000000, -0.000000000000000000, -0.000000000000000000 ) ) ;
#2161=CARTESIAN_POINT ( 'NONE',  ( -78.00000000000002842, 59.24264068711927678, 11.22792543327563131 ) ) ;
#2169=CARTESIAN_POINT ( 'NONE',  ( -78.00000000000002842, 42.27207793864211283, 12.72792543327562775 ) ) ;
#2179=DIRECTION ( 'NONE',  ( 0.000000000000000000, 1.000000000000000000, 0.000000000000000000 ) ) ;
#2183=EDGE_CURVE ( 'NONE', #6748, #6864, #10857, .T. ) ;
#2186=VERTEX_POINT ( 'NONE', #5477 ) ;
#2190=DIRECTION ( 'NONE',  ( 0.000000000000000000, 0.000000000000000000, 1.000000000000000000 ) ) ;
#2192=EDGE_CURVE ( 'NONE', #4978, #10867, #2886, .T. ) ;
#2193=EDGE_LOOP ( 'NONE', ( #828, #7872 ) ) ;
#2195=DIRECTION ( 'NONE',  ( -1.000000000000000000, -0.000000000000000000, -0.000000000000000000 ) ) ;
#2201=EDGE_CURVE ( 'NONE', #6484, #4456, #1918, .T. ) ;
#2204=ORIENTED_EDGE ( 'NONE', *, *, #3378, .F. ) ;
#2207=DIRECTION ( 'NONE',  ( -1.000000000000000000, -0.000000000000000000, -0.000000000000000000 ) ) ;
#2222=AXIS2_PLACEMENT_3D ( 'NONE', #3167, #7958, #9803 ) ;
#2227=ORIENTED_EDGE ( 'NONE', *, *, #9507, .F. ) ;
#2229=CARTESIAN_POINT ( 'NONE',  ( -80.00000000000002842, 46.51471862576140381, 3.371917798797308130E-06 ) ) ;
#2232=CARTESIAN_POINT ( 'NONE',  ( -78.00000000000001421, 71.97056274847716395, 3.371917795327861178E-06 ) ) ;
#2240=CARTESIAN_POINT ( 'NONE',  ( -80.00000000000001421, 59.24264068711927678, 2.742644059037073312 ) ) ;
#2246=ORIENTED_EDGE ( 'NONE', *, *, #797, .T. ) ;
#2250=LINE ( 'NONE', #330, #11759 ) ;
#2255=APPLICATION_CONTEXT ( 'automotive_design' ) ;
#2273=CYLINDRICAL_SURFACE ( 'NONE', #1561, 1.500000000000000444 ) ;
#2274=AXIS2_PLACEMENT_3D ( 'NONE', #1536, #9627, #6947 ) ;
#2275=DIRECTION ( 'NONE',  ( 0.000000000000000000, 1.000000000000000000, 0.000000000000000000 ) ) ;
#2277=CARTESIAN_POINT ( 'NONE',  ( -78.00000000000002842, 42.27207793864211283, 11.22792543327562775 ) ) ;
#2279=CARTESIAN_POINT ( 'NONE',  ( -78.00000000000002842, 38.02943725152282184, -1.499996628082202133 ) ) ;
#2286=EDGE_CURVE ( 'NONE', #5423, #10744, #2501, .T. ) ;
#2288=EDGE_CURVE ( 'NONE', #11145, #2349, #6247, .T. ) ;
#2294=ORIENTED_EDGE ( 'NONE', *, *, #5780, .T. ) ;
#2296=CARTESIAN_POINT ( 'NONE',  ( -78.00000000000001421, 54.99999999999998579, -8.485278002320759683 ) ) ;
#2299=CARTESIAN_POINT ( 'NONE',  ( -78.00000000000001421, 63.48528137423857487, -9.985278002320759683 ) ) ;
#2302=ORIENTED_EDGE ( 'NONE', *, *, #2342, .T. ) ;
#2303=DIRECTION ( 'NONE',  ( 0.000000000000000000, 0.000000000000000000, 1.000000000000000000 ) ) ;
#2305=CIRCLE ( 'NONE', #7289, 1.500000000000001332 ) ;
#2307=ORIENTED_EDGE ( 'NONE', *, *, #1685, .F. ) ;
#2329=DIRECTION ( 'NONE',  ( -1.000000000000000000, -0.000000000000000000, -0.000000000000000000 ) ) ;
#2334=EDGE_CURVE ( 'NONE', #1831, #8790, #6569, .T. ) ;
#2338=ORIENTED_EDGE ( 'NONE', *, *, #8504, .T. ) ;
#2341=DIRECTION ( 'NONE',  ( -1.000000000000000000, -0.000000000000000000, -0.000000000000000000 ) ) ;
#2342=EDGE_CURVE ( 'NONE', #6241, #11230, #5789, .T. ) ;
#2348=FACE_OUTER_BOUND ( 'NONE', #11660, .T. ) ;
#2349=VERTEX_POINT ( 'NONE', #2779 ) ;
#2352=DIRECTION ( 'NONE',  ( 0.000000000000000000, 1.000000000000000000, 0.000000000000000000 ) ) ;
#2353=EDGE_LOOP ( 'NONE', ( #10086, #5582, #6860, #5016 ) ) ;
#2363=VERTEX_POINT ( 'NONE', #8233 ) ;
#2364=CARTESIAN_POINT ( 'NONE',  ( -78.00000000000001421, 54.99999999999999289, -16.97055937655931501 ) ) ;
#2375=CARTESIAN_POINT ( 'NONE',  ( -80.00000000000002842, 50.75735931288069480, 4.242644059037076865 ) ) ;
#2384=VERTEX_POINT ( 'NONE', #9244 ) ;
#2386=DIRECTION ( 'NONE',  ( -1.000000000000000000, -0.000000000000000000, -0.000000000000000000 ) ) ;
#2391=CARTESIAN_POINT ( 'NONE',  ( -78.00000000000001421, 59.24264068711928388, -11.22791868944003824 ) ) ;
#2393=LINE ( 'NONE', #6068, #11623 ) ;
#2397=ADVANCED_FACE ( 'NONE', ( #8346 ), #130, .F. ) ;
#2399=CARTESIAN_POINT ( 'NONE',  ( -80.00000000000001421, 71.97056274847716395, -1.499996628082204797 ) ) ;
#2400=EDGE_LOOP ( 'NONE', ( #6141, #5251 ) ) ;
#2402=EDGE_LOOP ( 'NONE', ( #591, #1737 ) ) ;
#2406=DIRECTION ( 'NONE',  ( -1.000000000000000000, -0.000000000000000000, -0.000000000000000000 ) ) ;
#2409=DIRECTION ( 'NONE',  ( -1.000000000000000000, -0.000000000000000000, -0.000000000000000000 ) ) ;
#2415=VECTOR ( 'NONE', #6695, 1000.000000000000000 ) ;
#2416=EDGE_CURVE ( 'NONE', #10654, #69, #1093, .T. ) ;
#2417=CARTESIAN_POINT ( 'NONE',  ( -80.00000000000002842, 54.99999999999998579, 8.485284746156354529 ) ) ;
#2420=CYLINDRICAL_SURFACE ( 'NONE', #2995, 1.499999999999999556 ) ;
#2423=CARTESIAN_POINT ( 'NONE',  ( -78.00000000000002842, 42.27207793864211283, -2.742637315201478909 ) ) ;
#2424=ADVANCED_FACE ( 'NONE', ( #68 ), #11088, .F. ) ;
#2435=DIRECTION ( 'NONE',  ( -1.000000000000000000, -0.000000000000000000, -0.000000000000000000 ) ) ;
#2437=ORIENTED_EDGE ( 'NONE', *, *, #10541, .F. ) ;
#2439=CIRCLE ( 'NONE', #3392, 1.500000000000001332 ) ;
#2442=( GEOMETRIC_REPRESENTATION_CONTEXT ( 3 ) GLOBAL_UNCERTAINTY_ASSIGNED_CONTEXT ( ( #4959 ) ) GLOBAL_UNIT_ASSIGNED_CONTEXT ( ( #4474, #11033, #983 ) ) REPRESENTATION_CONTEXT ( 'NONE', 'WORKASPACE' ) );
#2443=VERTEX_POINT ( 'NONE', #10603 ) ;
#2451=CARTESIAN_POINT ( 'NONE',  ( -80.00000000000002842, 59.24264068711927678, 14.22792543327563131 ) ) ;
#2458=CARTESIAN_POINT ( 'NONE',  ( -78.00000000000002842, 46.51471862576140381, 9.985284746156354529 ) ) ;
#2462=DIRECTION ( 'NONE',  ( -1.000000000000000000, -0.000000000000000000, -0.000000000000000000 ) ) ;
#2463=EDGE_LOOP ( 'NONE', ( #3668, #6876 ) ) ;
#2480=EDGE_CURVE ( 'NONE', #6241, #1033, #2305, .T. ) ;
#2481=CARTESIAN_POINT ( 'NONE',  ( -80.00000000000000000, 55.00000000000000000, -21.50000000000000000 ) ) ;
#2483=CIRCLE ( 'NONE', #8034, 1.500000000000001332 ) ;
#2485=AXIS2_PLACEMENT_3D ( 'NONE', #102, #7322, #8321 ) ;
#2487=ORIENTED_EDGE ( 'NONE', *, *, #3740, .T. ) ;
#2488=DIRECTION ( 'NONE',  ( 0.000000000000000000, 0.000000000000000000, 1.000000000000000000 ) ) ;
#2489=CARTESIAN_POINT ( 'NONE',  ( -78.00000000000001421, 63.48528137423857487, 8.485284746156350977 ) ) ;
#2494=AXIS2_PLACEMENT_3D ( 'NONE', #8818, #2462, #8757 ) ;
#2495=ORIENTED_EDGE ( 'NONE', *, *, #4330, .T. ) ;
#2500=EDGE_CURVE ( 'NONE', #1770, #69, #9008, .T. ) ;
#2501=CIRCLE ( 'NONE', #2698, 1.500000000000001332 ) ;
#2505=EDGE_LOOP ( 'NONE', ( #5491, #4064 ) ) ;
#2507=CIRCLE ( 'NONE', #10717, 1.500000000000001332 ) ;
#2508=CARTESIAN_POINT ( 'NONE',  ( -80.00000000000002842, 54.99999999999998579, 16.97056612039490986 ) ) ;
#2514=EDGE_LOOP ( 'NONE', ( #3420, #232 ) ) ;
#2523=DIRECTION ( 'NONE',  ( -1.000000000000000000, -0.000000000000000000, -0.000000000000000000 ) ) ;
#2525=CARTESIAN_POINT ( 'NONE',  ( -78.00000000000002842, 50.75735931288069480, 12.72792543327563131 ) ) ;
#2527=DIRECTION ( 'NONE',  ( -1.000000000000000000, -0.000000000000000000, -0.000000000000000000 ) ) ;
#2528=VERTEX_POINT ( 'NONE', #1687 ) ;
#2530=ORIENTED_EDGE ( 'NONE', *, *, #5259, .F. ) ;
#2537=CARTESIAN_POINT ( 'NONE',  ( -78.00000000000002842, 42.27207793864211283, 2.742644059037075976 ) ) ;
#2545=CARTESIAN_POINT ( 'NONE',  ( -78.00000000000002842, 46.51471862576140381, 3.371917798797308130E-06 ) ) ;
#2554=EDGE_CURVE ( 'NONE', #9492, #1807, #7105, .T. ) ;
#2557=DIRECTION ( 'NONE',  ( -1.000000000000000000, -0.000000000000000000, -0.000000000000000000 ) ) ;
#2563=DIRECTION ( 'NONE',  ( -1.000000000000000000, -0.000000000000000000, -0.000000000000000000 ) ) ;
#2566=DIRECTION ( 'NONE',  ( 0.000000000000000000, 1.000000000000000000, 0.000000000000000000 ) ) ;
#2569=DIRECTION ( 'NONE',  ( 0.000000000000000000, 0.000000000000000000, -1.000000000000000000 ) ) ;
#2574=EDGE_CURVE ( 'NONE', #656, #3299, #5189, .T. ) ;
#2587=CARTESIAN_POINT ( 'NONE',  ( -78.00000000000001421, 67.72792206135787296, 4.242644059037073312 ) ) ;
#2606=EDGE_LOOP ( 'NONE', ( #6377, #11266 ) ) ;
#2610=VERTEX_POINT ( 'NONE', #10169 ) ;
#2614=CARTESIAN_POINT ( 'NONE',  ( -80.00000000000002842, 42.27207793864211283, -4.242637315201479353 ) ) ;
#2625=ORIENTED_EDGE ( 'NONE', *, *, #9797, .F. ) ;
#2630=AXIS2_PLACEMENT_3D ( 'NONE', #1301, #6948, #10456 ) ;
#2637=CARTESIAN_POINT ( 'NONE',  ( -78.00000000000002842, 42.27207793864211283, 12.72792543327562775 ) ) ;
#2643=VERTEX_POINT ( 'NONE', #2148 ) ;
#2648=DIRECTION ( 'NONE',  ( -1.000000000000000000, -0.000000000000000000, -0.000000000000000000 ) ) ;
#2649=AXIS2_PLACEMENT_3D ( 'NONE', #10829, #4493, #1611 ) ;
#2669=CIRCLE ( 'NONE', #7273, 1.500000000000001332 ) ;
#2670=CIRCLE ( 'NONE', #362, 1.500000000000001332 ) ;
#2674=FILL_AREA_STYLE ('',( #1816 ) ) ;
#2683=CARTESIAN_POINT ( 'NONE',  ( -78.00000000000001421, 67.72792206135787296, -11.22791868944004534 ) ) ;
#2685=CYLINDRICAL_SURFACE ( 'NONE', #4988, 1.500000000000001332 ) ;
#2690=AXIS2_PLACEMENT_3D ( 'NONE', #5697, #5452, #9271 ) ;
#2693=EDGE_CURVE ( 'NONE', #11779, #3307, #4608, .T. ) ;
#2694=VECTOR ( 'NONE', #615, 1000.000000000000000 ) ;
#2698=AXIS2_PLACEMENT_3D ( 'NONE', #2960, #1031, #3679 ) ;
#2710=EDGE_CURVE ( 'NONE', #9787, #3028, #4226, .T. ) ;
#2718=DIRECTION ( 'NONE',  ( 0.000000000000000000, 0.000000000000000000, 1.000000000000000000 ) ) ;
#2733=EDGE_LOOP ( 'NONE', ( #5220, #4348, #8989, #5133 ) ) ;
#2734=ADVANCED_FACE ( 'NONE', ( #9515 ), #7668, .F. ) ;
#2738=CARTESIAN_POINT ( 'NONE',  ( -78.00000000000002842, 54.99999999999998579, 16.97056612039490986 ) ) ;
#2754=DIRECTION ( 'NONE',  ( -1.000000000000000000, -0.000000000000000000, -0.000000000000000000 ) ) ;
#2766=DIRECTION ( 'NONE',  ( 0.000000000000000000, 1.000000000000000000, 0.000000000000000000 ) ) ;
#2772=CARTESIAN_POINT ( 'NONE',  ( -80.00000000000001421, 67.72792206135787296, 12.72792543327562775 ) ) ;
#2779=CARTESIAN_POINT ( 'NONE',  ( -78.00000000000001421, 46.51471862576140381, -6.985278002320760571 ) ) ;
#2784=ORIENTED_EDGE ( 'NONE', *, *, #11012, .T. ) ;
#2792=ORIENTED_EDGE ( 'NONE', *, *, #4925, .T. ) ;
#2795=DIRECTION ( 'NONE',  ( -1.000000000000000000, -0.000000000000000000, -0.000000000000000000 ) ) ;
#2797=AXIS2_PLACEMENT_3D ( 'NONE', #5899, #4998, #2352 ) ;
#2799=FACE_OUTER_BOUND ( 'NONE', #5343, .T. ) ;
#2801=ORIENTED_EDGE ( 'NONE', *, *, #5075, .T. ) ;
#2810=CARTESIAN_POINT ( 'NONE',  ( -78.00000000000000000, 54.99999999999999289, -1.499996628082203021 ) ) ;
#2813=VERTEX_POINT ( 'NONE', #6656 ) ;
#2818=CIRCLE ( 'NONE', #3578, 1.500000000000001332 ) ;
#2823=AXIS2_PLACEMENT_3D ( 'NONE', #2545, #6272, #7168 ) ;
#2827=DIRECTION ( 'NONE',  ( -1.000000000000000000, -0.000000000000000000, -0.000000000000000000 ) ) ;
#2835=DIRECTION ( 'NONE',  ( 0.000000000000000000, 0.000000000000000000, 1.000000000000000000 ) ) ;
#2843=SURFACE_STYLE_USAGE ( .BOTH. , #3739 ) ;
#2849=VERTEX_POINT ( 'NONE', #7071 ) ;
#2853=DIRECTION ( 'NONE',  ( 0.000000000000000000, 1.000000000000000000, 0.000000000000000000 ) ) ;
#2854=FACE_OUTER_BOUND ( 'NONE', #9476, .T. ) ;
#2855=LINE ( 'NONE', #10154, #11835 ) ;
#2856=LINE ( 'NONE', #10155, #4222 ) ;
#2857=ADVANCED_FACE ( 'NONE', ( #1542 ), #8738, .F. ) ;
#2862=VECTOR ( 'NONE', #4716, 1000.000000000000000 ) ;
#2865=DIRECTION ( 'NONE',  ( 0.000000000000000000, 1.000000000000000000, 0.000000000000000000 ) ) ;
#2874=DIRECTION ( 'NONE',  ( 0.000000000000000000, 1.000000000000000000, 0.000000000000000000 ) ) ;
#2881=CARTESIAN_POINT ( 'NONE',  ( -78.00000000000000000, 55.00000000000000000, -21.50000000000000000 ) ) ;
#2886=CIRCLE ( 'NONE', #10134, 1.500000000000001332 ) ;
#2889=AXIS2_PLACEMENT_3D ( 'NONE', #8039, #1617, #6195 ) ;
#2893=FACE_BOUND ( 'NONE', #11128, .T. ) ;
#2899=EDGE_LOOP ( 'NONE', ( #2307, #2246, #10517, #5763 ) ) ;
#2901=DIRECTION ( 'NONE',  ( -1.000000000000000000, -0.000000000000000000, -0.000000000000000000 ) ) ;
#2916=EDGE_LOOP ( 'NONE', ( #7440, #8269 ) ) ;
#2922=EDGE_CURVE ( 'NONE', #3229, #8790, #11582, .T. ) ;
#2923=ORIENTED_EDGE ( 'NONE', *, *, #6293, .T. ) ;
#2927=DIRECTION ( 'NONE',  ( 0.000000000000000000, 0.000000000000000000, 1.000000000000000000 ) ) ;
#2931=CARTESIAN_POINT ( 'NONE',  ( -80.00000000000001421, 67.72792206135787296, 4.242644059037073312 ) ) ;
#2932=DIRECTION ( 'NONE',  ( -1.000000000000000000, -0.000000000000000000, -0.000000000000000000 ) ) ;
#2933=CARTESIAN_POINT ( 'NONE',  ( -78.00000000000002842, 46.51471862576140381, 3.371917798797308130E-06 ) ) ;
#2937=EDGE_CURVE ( 'NONE', #4386, #932, #7392, .T. ) ;
#2951=DIRECTION ( 'NONE',  ( 0.000000000000000000, 0.000000000000000000, 1.000000000000000000 ) ) ;
#2954=CYLINDRICAL_SURFACE ( 'NONE', #938, 1.500000000000000444 ) ;
#2960=CARTESIAN_POINT ( 'NONE',  ( -78.00000000000002842, 46.51471862576140381, 8.485284746156354529 ) ) ;
#2964=CARTESIAN_POINT ( 'NONE',  ( -80.00000000000002842, 54.99999999999998579, 16.97056612039490986 ) ) ;
#2977=CARTESIAN_POINT ( 'NONE',  ( -80.00000000000001421, 67.72792206135787296, -2.742637315201482462 ) ) ;
#2989=DIRECTION ( 'NONE',  ( 0.000000000000000000, 1.000000000000000000, 0.000000000000000000 ) ) ;
#2992=CARTESIAN_POINT ( 'NONE',  ( -78.00000000000002842, 42.27207793864211283, 4.242644059037075976 ) ) ;
#2995=AXIS2_PLACEMENT_3D ( 'NONE', #9842, #6091, #3374 ) ;
#2998=EDGE_LOOP ( 'NONE', ( #8210, #9411, #7687, #773 ) ) ;
#3005=ORIENTED_EDGE ( 'NONE', *, *, #1557, .F. ) ;
#3008=CARTESIAN_POINT ( 'NONE',  ( -80.00000000000001421, 46.51471862576140381, -6.985278002320760571 ) ) ;
#3009=DIRECTION ( 'NONE',  ( 0.000000000000000000, 0.000000000000000000, 1.000000000000000000 ) ) ;
#3013=AXIS2_PLACEMENT_3D ( 'NONE', #4907, #8732, #7724 ) ;
#3014=CARTESIAN_POINT ( 'NONE',  ( -80.00000000000001421, 42.27207793864211283, -11.22791868944003824 ) ) ;
#3017=FACE_OUTER_BOUND ( 'NONE', #9790, .T. ) ;
#3018=CARTESIAN_POINT ( 'NONE',  ( -78.00000000000001421, 59.24264068711927678, -4.242637315201482906 ) ) ;
#3023=CIRCLE ( 'NONE', #1097, 1.500000000000001332 ) ;
#3027=CARTESIAN_POINT ( 'NONE',  ( -78.00000000000001421, 54.99999999999999289, -18.47055937655931501 ) ) ;
#3028=VERTEX_POINT ( 'NONE', #6648 ) ;
#3032=ORIENTED_EDGE ( 'NONE', *, *, #5297, .T. ) ;
#3035=CARTESIAN_POINT ( 'NONE',  ( -78.00000000000001421, 67.72792206135787296, 5.742644059037073312 ) ) ;
#3039=ORIENTED_EDGE ( 'NONE', *, *, #4619, .F. ) ;
#3040=ADVANCED_FACE ( 'NONE', ( #5867 ), #5992, .F. ) ;
#3043=DIRECTION ( 'NONE',  ( -1.000000000000000000, -0.000000000000000000, -0.000000000000000000 ) ) ;
#3044=AXIS2_PLACEMENT_3D ( 'NONE', #11362, #4915, #5939 ) ;
#3049=CARTESIAN_POINT ( 'NONE',  ( -78.00000000000001421, 63.48528137423857487, 8.485284746156350977 ) ) ;
#3055=ORIENTED_EDGE ( 'NONE', *, *, #2693, .T. ) ;
#3057=AXIS2_PLACEMENT_3D ( 'NONE', #4248, #6232, #6956 ) ;
#3064=DIRECTION ( 'NONE',  ( 0.000000000000000000, 0.000000000000000000, 1.000000000000000000 ) ) ;
#3072=EDGE_CURVE ( 'NONE', #11556, #4778, #11195, .T. ) ;
#3074=AXIS2_PLACEMENT_3D ( 'NONE', #2933, #881, #5636 ) ;
#3076=DIRECTION ( 'NONE',  ( -1.000000000000000000, -0.000000000000000000, -0.000000000000000000 ) ) ;
#3077=ORIENTED_EDGE ( 'NONE', *, *, #3309, .F. ) ;
#3091=ORIENTED_EDGE ( 'NONE', *, *, #10975, .F. ) ;
#3099=AXIS2_PLACEMENT_3D ( 'NONE', #10764, #9152, #5393 ) ;
#3102=CARTESIAN_POINT ( 'NONE',  ( -78.00000000000001421, 67.72792206135787296, 12.72792543327562775 ) ) ;
#3103=EDGE_CURVE ( 'NONE', #2643, #9669, #10453, .T. ) ;
#3109=DIRECTION ( 'NONE',  ( 0.000000000000000000, 1.000000000000000000, 0.000000000000000000 ) ) ;
#3140=AXIS2_PLACEMENT_3D ( 'NONE', #7132, #2563, #3517 ) ;
#3141=LINE ( 'NONE', #2056, #6714 ) ;
#3145=ORIENTED_EDGE ( 'NONE', *, *, #3317, .T. ) ;
#3153=DIRECTION ( 'NONE',  ( -1.000000000000000000, -0.000000000000000000, -0.000000000000000000 ) ) ;
#3161=CARTESIAN_POINT ( 'NONE',  ( -78.00000000000001421, 67.72792206135787296, -14.22791868944004356 ) ) ;
#3164=ORIENTED_EDGE ( 'NONE', *, *, #1682, .F. ) ;
#3167=CARTESIAN_POINT ( 'NONE',  ( -78.00000000000001421, 67.72792206135787296, 12.72792543327562775 ) ) ;
#3176=ORIENTED_EDGE ( 'NONE', *, *, #6074, .T. ) ;
#3181=ORIENTED_EDGE ( 'NONE', *, *, #10879, .F. ) ;
#3187=EDGE_CURVE ( 'NONE', #6484, #1706, #8968, .T. ) ;
#3197=DIRECTION ( 'NONE',  ( -1.000000000000000000, -0.000000000000000000, -0.000000000000000000 ) ) ;
#3202=ORIENTED_EDGE ( 'NONE', *, *, #1871, .T. ) ;
#3203=LINE ( 'NONE', #1468, #9891 ) ;
#3212=DIRECTION ( 'NONE',  ( 0.000000000000000000, 1.000000000000000000, 0.000000000000000000 ) ) ;
#3214=ORIENTED_EDGE ( 'NONE', *, *, #3934, .F. ) ;
#3221=VERTEX_POINT ( 'NONE', #4174 ) ;
#3229=VERTEX_POINT ( 'NONE', #3273 ) ;
#3230=DIRECTION ( 'NONE',  ( 0.000000000000000000, 0.000000000000000000, 1.000000000000000000 ) ) ;
#3231=CARTESIAN_POINT ( 'NONE',  ( -78.00000000000000000, 55.00000000000000000, 0.000000000000000000 ) ) ;
#3238=ORIENTED_EDGE ( 'NONE', *, *, #9059, .F. ) ;
#3240=AXIS2_PLACEMENT_3D ( 'NONE', #7333, #8333, #8465 ) ;
#3250=CIRCLE ( 'NONE', #4210, 1.500000000000001332 ) ;
#3261=CIRCLE ( 'NONE', #6367, 1.500000000000001332 ) ;
#3269=CARTESIAN_POINT ( 'NONE',  ( -80.00000000000001421, 71.97056274847716395, 3.371917795327861178E-06 ) ) ;
#3273=CARTESIAN_POINT ( 'NONE',  ( -80.00000000000002842, 54.99999999999998579, 15.47056612039490986 ) ) ;
#3274=EDGE_CURVE ( 'NONE', #11230, #1850, #6630, .T. ) ;
#3282=AXIS2_PLACEMENT_3D ( 'NONE', #6063, #758, #1725 ) ;
#3287=LINE ( 'NONE', #8977, #5352 ) ;
#3291=FACE_BOUND ( 'NONE', #4819, .T. ) ;
#3299=VERTEX_POINT ( 'NONE', #10572 ) ;
#3300=DIRECTION ( 'NONE',  ( -1.000000000000000000, -0.000000000000000000, -0.000000000000000000 ) ) ;
#3304=ORIENTED_EDGE ( 'NONE', *, *, #9157, .T. ) ;
#3305=DIRECTION ( 'NONE',  ( -1.000000000000000000, -0.000000000000000000, -0.000000000000000000 ) ) ;
#3307=VERTEX_POINT ( 'NONE', #6046 ) ;
#3309=EDGE_CURVE ( 'NONE', #11604, #8631, #9678, .T. ) ;
#3311=CARTESIAN_POINT ( 'NONE',  ( -78.00000000000002842, 50.75735931288069480, 12.72792543327563131 ) ) ;
#3317=EDGE_CURVE ( 'NONE', #3221, #5447, #4516, .T. ) ;
#3318=LINE ( 'NONE', #6985, #11504 ) ;
#3321=CARTESIAN_POINT ( 'NONE',  ( -78.00000000000001421, 67.72792206135787296, -4.242637315201482906 ) ) ;
#3329=EDGE_LOOP ( 'NONE', ( #10951, #3164, #782, #8582 ) ) ;
#3332=VECTOR ( 'NONE', #5999, 1000.000000000000000 ) ;
#3336=ORIENTED_EDGE ( 'NONE', *, *, #10323, .F. ) ;
#3340=LINE ( 'NONE', #1599, #9731 ) ;
#3351=VECTOR ( 'NONE', #1109, 1000.000000000000000 ) ;
#3353=DIRECTION ( 'NONE',  ( 0.000000000000000000, 0.000000000000000000, 1.000000000000000000 ) ) ;
#3364=CIRCLE ( 'NONE', #4906, 1.500000000000001332 ) ;
#3370=EDGE_CURVE ( 'NONE', #9755, #5641, #3364, .T. ) ;
#3371=CARTESIAN_POINT ( 'NONE',  ( -78.00000000000000000, 55.00000000000000000, 21.50000000000000000 ) ) ;
#3374=DIRECTION ( 'NONE',  ( 0.000000000000000000, 0.000000000000000000, 1.000000000000000000 ) ) ;
#3375=CIRCLE ( 'NONE', #8550, 1.500000000000001332 ) ;
#3378=EDGE_CURVE ( 'NONE', #2186, #9436, #861, .T. ) ;
#3380=EDGE_LOOP ( 'NONE', ( #7030, #10926 ) ) ;
#3384=CIRCLE ( 'NONE', #8755, 1.500000000000001332 ) ;
#3392=AXIS2_PLACEMENT_3D ( 'NONE', #2232, #6139, #7873 ) ;
#3396=ORIENTED_EDGE ( 'NONE', *, *, #804, .F. ) ;
#3403=ORIENTED_EDGE ( 'NONE', *, *, #1765, .F. ) ;
#3407=AXIS2_PLACEMENT_3D ( 'NONE', #7024, #5160, #1320 ) ;
#3414=CARTESIAN_POINT ( 'NONE',  ( -78.00000000000001421, 50.75735931288069480, -12.72791868944003824 ) ) ;
#3417=EDGE_LOOP ( 'NONE', ( #3620, #10218, #1602, #3403 ) ) ;
#3419=CARTESIAN_POINT ( 'NONE',  ( -78.00000000000002842, 59.24264068711927678, 14.22792543327563131 ) ) ;
#3420=ORIENTED_EDGE ( 'NONE', *, *, #10995, .T. ) ;
#3449=EDGE_CURVE ( 'NONE', #3299, #656, #6436, .T. ) ;
#3455=ORIENTED_EDGE ( 'NONE', *, *, #8368, .T. ) ;
#3456=VECTOR ( 'NONE', #11025, 1000.000000000000000 ) ;
#3459=FACE_OUTER_BOUND ( 'NONE', #5941, .T. ) ;
#3463=EDGE_CURVE ( 'NONE', #4456, #11337, #4100, .T. ) ;
#3465=CIRCLE ( 'NONE', #7321, 1.500000000000001332 ) ;
#3471=EDGE_LOOP ( 'NONE', ( #2011, #5130 ) ) ;
#3473=CARTESIAN_POINT ( 'NONE',  ( -78.00000000000001421, 67.72792206135787296, 12.72792543327562775 ) ) ;
#3474=DIRECTION ( 'NONE',  ( -1.000000000000000000, -0.000000000000000000, -0.000000000000000000 ) ) ;
#3485=ORIENTED_EDGE ( 'NONE', *, *, #9157, .F. ) ;
#3494=VERTEX_POINT ( 'NONE', #2240 ) ;
#3501=EDGE_LOOP ( 'NONE', ( #6121, #3561, #7296, #7759 ) ) ;
#3517=DIRECTION ( 'NONE',  ( 0.000000000000000000, 1.000000000000000000, 0.000000000000000000 ) ) ;
#3523=FACE_OUTER_BOUND ( 'NONE', #334, .T. ) ;
#3551=EDGE_CURVE ( 'NONE', #849, #1312, #7026, .T. ) ;
#3552=LINE ( 'NONE', #7223, #3926 ) ;
#3558=ORIENTED_EDGE ( 'NONE', *, *, #1152, .F. ) ;
#3561=ORIENTED_EDGE ( 'NONE', *, *, #6847, .T. ) ;
#3570=CIRCLE ( 'NONE', #9491, 1.500000000000001332 ) ;
#3571=DIRECTION ( 'NONE',  ( 0.000000000000000000, 0.000000000000000000, 1.000000000000000000 ) ) ;
#3578=AXIS2_PLACEMENT_3D ( 'NONE', #6476, #11060, #2989 ) ;
#3580=FACE_OUTER_BOUND ( 'NONE', #326, .T. ) ;
#3586=CIRCLE ( 'NONE', #6459, 1.500000000000001332 ) ;
#3587=VERTEX_POINT ( 'NONE', #442 ) ;
#3589=STYLED_ITEM ( 'NONE', ( #202 ), #1113 ) ;
#3597=DIRECTION ( 'NONE',  ( 0.000000000000000000, 1.000000000000000000, 0.000000000000000000 ) ) ;
#3606=CYLINDRICAL_SURFACE ( 'NONE', #7050, 21.50000000000000000 ) ;
#3607=ORIENTED_EDGE ( 'NONE', *, *, #6827, .T. ) ;
#3618=ORIENTED_EDGE ( 'NONE', *, *, #9071, .T. ) ;
#3620=ORIENTED_EDGE ( 'NONE', *, *, #3551, .F. ) ;
#3625=ORIENTED_EDGE ( 'NONE', *, *, #6915, .F. ) ;
#3628=ORIENTED_EDGE ( 'NONE', *, *, #2500, .F. ) ;
#3635=CARTESIAN_POINT ( 'NONE',  ( -78.00000000000001421, 67.72792206135787296, -4.242637315201482906 ) ) ;
#3637=DIRECTION ( 'NONE',  ( -1.000000000000000000, -0.000000000000000000, -0.000000000000000000 ) ) ;
#3641=DIRECTION ( 'NONE',  ( -1.000000000000000000, -0.000000000000000000, -0.000000000000000000 ) ) ;
#3644=AXIS2_PLACEMENT_3D ( 'NONE', #6082, #548, #4039 ) ;
#3645=EDGE_CURVE ( 'NONE', #430, #723, #11217, .T. ) ;
#3646=CARTESIAN_POINT ( 'NONE',  ( -80.00000000000002842, 50.75735931288069480, 11.22792543327563131 ) ) ;
#3652=AXIS2_PLACEMENT_3D ( 'NONE', #781, #5353, #10726 ) ;
#3653=CARTESIAN_POINT ( 'NONE',  ( -78.00000000000002842, 54.99999999999998579, 18.47056612039490986 ) ) ;
#3656=CARTESIAN_POINT ( 'NONE',  ( -80.00000000000001421, 54.99999999999998579, -8.485278002320759683 ) ) ;
#3657=ORIENTED_EDGE ( 'NONE', *, *, #8008, .T. ) ;
#3668=ORIENTED_EDGE ( 'NONE', *, *, #9507, .T. ) ;
#3671=DIRECTION ( 'NONE',  ( 0.000000000000000000, 0.000000000000000000, 1.000000000000000000 ) ) ;
#3675=CIRCLE ( 'NONE', #7294, 1.500000000000001332 ) ;
#3679=DIRECTION ( 'NONE',  ( 0.000000000000000000, 1.000000000000000000, 0.000000000000000000 ) ) ;
#3689=DIRECTION ( 'NONE',  ( 0.000000000000000000, 1.000000000000000000, 0.000000000000000000 ) ) ;
#3698=ORIENTED_EDGE ( 'NONE', *, *, #4340, .F. ) ;
#3703=LINE ( 'NONE', #7430, #10067 ) ;
#3715=SHAPE_REPRESENTATION ( 'perforated grinding plate', ( #4738 ), #2442 ) ;
#3721=ORIENTED_EDGE ( 'NONE', *, *, #798, .T. ) ;
#3729=ORIENTED_EDGE ( 'NONE', *, *, #6830, .F. ) ;
#3732=CARTESIAN_POINT ( 'NONE',  ( -78.00000000000001421, 42.27207793864211283, -12.72791868944003824 ) ) ;
#3739=SURFACE_SIDE_STYLE ('',( #7407 ) ) ;
#3740=EDGE_CURVE ( 'NONE', #10654, #9231, #6637, .T. ) ;
#3751=EDGE_CURVE ( 'NONE', #2443, #241, #5302, .T. ) ;
#3752=AXIS2_PLACEMENT_3D ( 'NONE', #10313, #4817, #5785 ) ;
#3776=CIRCLE ( 'NONE', #9123, 1.500000000000001332 ) ;
#3781=CIRCLE ( 'NONE', #895, 1.500000000000001332 ) ;
#3785=CARTESIAN_POINT ( 'NONE',  ( -78.00000000000002842, 46.51471862576140381, 8.485284746156354529 ) ) ;
#3786=FACE_BOUND ( 'NONE', #11441, .T. ) ;
#3789=CIRCLE ( 'NONE', #3407, 1.500000000000001332 ) ;
#3795=ADVANCED_FACE ( 'NONE', ( #6208 ), #2420, .F. ) ;
#3796=ORIENTED_EDGE ( 'NONE', *, *, #2416, .F. ) ;
#3812=EDGE_CURVE ( 'NONE', #4662, #723, #4524, .T. ) ;
#3816=DIRECTION ( 'NONE',  ( -1.000000000000000000, -0.000000000000000000, -0.000000000000000000 ) ) ;
#3826=AXIS2_PLACEMENT_3D ( 'NONE', #6130, #6072, #11552 ) ;
#3832=UNCERTAINTY_MEASURE_WITH_UNIT (LENGTH_MEASURE( 1.000000000000000082E-05 ), #11105, 'distance_accuracy_value', 'NONE');
#3844=AXIS2_PLACEMENT_3D ( 'NONE', #2489, #1757, #8119 ) ;
#3846=ORIENTED_EDGE ( 'NONE', *, *, #3812, .T. ) ;
#3848=AXIS2_PLACEMENT_3D ( 'NONE', #4753, #247, #6800 ) ;
#3850=DIRECTION ( 'NONE',  ( -1.000000000000000000, -0.000000000000000000, -0.000000000000000000 ) ) ;
#3855=CIRCLE ( 'NONE', #1366, 1.500000000000001332 ) ;
#3866=AXIS2_PLACEMENT_3D ( 'NONE', #2417, #4278, #6870 ) ;
#3867=CARTESIAN_POINT ( 'NONE',  ( -80.00000000000001421, 54.99999999999999289, -16.97055937655931501 ) ) ;
#3878=DIRECTION ( 'NONE',  ( -1.000000000000000000, -0.000000000000000000, -0.000000000000000000 ) ) ;
#3886=DIRECTION ( 'NONE',  ( 0.000000000000000000, 1.000000000000000000, 0.000000000000000000 ) ) ;
#3888=EDGE_LOOP ( 'NONE', ( #6818, #10413 ) ) ;
#3891=EDGE_CURVE ( 'NONE', #10599, #3494, #5382, .T. ) ;
#3898=ORIENTED_EDGE ( 'NONE', *, *, #798, .F. ) ;
#3903=DIRECTION ( 'NONE',  ( 0.000000000000000000, 1.000000000000000000, 0.000000000000000000 ) ) ;
#3908=DIRECTION ( 'NONE',  ( -1.000000000000000000, -0.000000000000000000, -0.000000000000000000 ) ) ;
#3909=FACE_BOUND ( 'NONE', #4530, .T. ) ;
#3913=ORIENTED_EDGE ( 'NONE', *, *, #6177, .T. ) ;
#3920=CARTESIAN_POINT ( 'NONE',  ( -80.00000000000001421, 71.97056274847716395, 1.500003371917795425 ) ) ;
#3926=VECTOR ( 'NONE', #10850, 1000.000000000000000 ) ;
#3929=EDGE_LOOP ( 'NONE', ( #1758, #3898 ) ) ;
#3932=DIRECTION ( 'NONE',  ( 0.000000000000000000, 1.000000000000000000, 0.000000000000000000 ) ) ;
#3934=EDGE_CURVE ( 'NONE', #3307, #11779, #9022, .T. ) ;
#3935=CARTESIAN_POINT ( 'NONE',  ( -78.00000000000002842, 42.27207793864211283, -4.242637315201479353 ) ) ;
#3937=EDGE_LOOP ( 'NONE', ( #6150, #4696, #10836, #4364 ) ) ;
#3939=CARTESIAN_POINT ( 'NONE',  ( -78.00000000000002842, 46.51471862576140381, 8.485284746156354529 ) ) ;
#3940=FACE_OUTER_BOUND ( 'NONE', #9972, .T. ) ;
#3946=CIRCLE ( 'NONE', #2797, 1.500000000000001332 ) ;
#3950=DIRECTION ( 'NONE',  ( 0.000000000000000000, 1.000000000000000000, 0.000000000000000000 ) ) ;
#3956=ORIENTED_EDGE ( 'NONE', *, *, #5685, .F. ) ;
#3965=VERTEX_POINT ( 'NONE', #1334 ) ;
#3995=DIRECTION ( 'NONE',  ( 0.000000000000000000, 1.000000000000000000, 0.000000000000000000 ) ) ;
#3997=CYLINDRICAL_SURFACE ( 'NONE', #6900, 1.500000000000000000 ) ;
#4011=LINE ( 'NONE', #2810, #10644 ) ;
#4018=CARTESIAN_POINT ( 'NONE',  ( -80.00000000000001421, 59.24264068711928388, -12.72791868944003824 ) ) ;
#4019=CIRCLE ( 'NONE', #5543, 1.500000000000001332 ) ;
#4025=AXIS2_PLACEMENT_3D ( 'NONE', #9147, #994, #2566 ) ;
#4026=ORIENTED_EDGE ( 'NONE', *, *, #6036, .F. ) ;
#4033=VECTOR ( 'NONE', #2113, 1000.000000000000000 ) ;
#4036=EDGE_LOOP ( 'NONE', ( #9975, #8707 ) ) ;
#4038=CIRCLE ( 'NONE', #8241, 1.500000000000001332 ) ;
#4039=DIRECTION ( 'NONE',  ( 0.000000000000000000, 1.000000000000000000, 0.000000000000000000 ) ) ;
#4047=VECTOR ( 'NONE', #3908, 1000.000000000000000 ) ;
#4064=ORIENTED_EDGE ( 'NONE', *, *, #4089, .T. ) ;
#4072=CARTESIAN_POINT ( 'NONE',  ( -78.00000000000001421, 54.99999999999999289, -18.47055937655931501 ) ) ;
#4076=ORIENTED_EDGE ( 'NONE', *, *, #10279, .F. ) ;
#4082=ORIENTED_EDGE ( 'NONE', *, *, #6074, .F. ) ;
#4089=EDGE_CURVE ( 'NONE', #3028, #9787, #4234, .T. ) ;
#4095=VECTOR ( 'NONE', #2329, 1000.000000000000000 ) ;
#4098=DIRECTION ( 'NONE',  ( -1.000000000000000000, -0.000000000000000000, -0.000000000000000000 ) ) ;
#4100=LINE ( 'NONE', #6811, #874 ) ;
#4101=EDGE_LOOP ( 'NONE', ( #4706, #11773, #10349, #3607 ) ) ;
#4102=CARTESIAN_POINT ( 'NONE',  ( -78.00000000000002842, 38.02943725152282184, 3.371917797929946392E-06 ) ) ;
#4105=ORIENTED_EDGE ( 'NONE', *, *, #5780, .F. ) ;
#4108=DIRECTION ( 'NONE',  ( 0.000000000000000000, 1.000000000000000000, 0.000000000000000000 ) ) ;
#4115=DIRECTION ( 'NONE',  ( 0.000000000000000000, 1.000000000000000000, 0.000000000000000000 ) ) ;
#4116=DIRECTION ( 'NONE',  ( -1.000000000000000000, -0.000000000000000000, -0.000000000000000000 ) ) ;
#4118=ORIENTED_EDGE ( 'NONE', *, *, #2922, .F. ) ;
#4128=PLANE ( 'NONE',  #2094 ) ;
#4130=AXIS2_PLACEMENT_3D ( 'NONE', #3939, #2195, #7545 ) ;
#4133=DIRECTION ( 'NONE',  ( 0.000000000000000000, 0.000000000000000000, 1.000000000000000000 ) ) ;
#4137=LINE ( 'NONE', #2279, #1828 ) ;
#4142=ORIENTED_EDGE ( 'NONE', *, *, #1460, .F. ) ;
#4151=ORIENTED_EDGE ( 'NONE', *, *, #11054, .T. ) ;
#4162=EDGE_CURVE ( 'NONE', #8007, #4492, #5978, .T. ) ;
#4171=ORIENTED_EDGE ( 'NONE', *, *, #6906, .T. ) ;
#4174=CARTESIAN_POINT ( 'NONE',  ( -80.00000000000002842, 59.24264068711927678, 11.22792543327563131 ) ) ;
#4178=CARTESIAN_POINT ( 'NONE',  ( -78.00000000000002842, 50.75735931288069480, 14.22792543327563131 ) ) ;
#4201=DIRECTION ( 'NONE',  ( 0.000000000000000000, 1.000000000000000000, 0.000000000000000000 ) ) ;
#4203=LINE ( 'NONE', #7862, #10893 ) ;
#4204=CIRCLE ( 'NONE', #10883, 1.500000000000001332 ) ;
#4210=AXIS2_PLACEMENT_3D ( 'NONE', #5164, #6911, #8699 ) ;
#4214=ORIENTED_EDGE ( 'NONE', *, *, #9599, .T. ) ;
#4217=CIRCLE ( 'NONE', #6341, 1.500000000000001332 ) ;
#4222=VECTOR ( 'NONE', #1954, 1000.000000000000000 ) ;
#4226=CIRCLE ( 'NONE', #7681, 1.500000000000001332 ) ;
#4234=CIRCLE ( 'NONE', #9959, 1.500000000000001332 ) ;
#4235=ORIENTED_EDGE ( 'NONE', *, *, #6504, .T. ) ;
#4248=CARTESIAN_POINT ( 'NONE',  ( -78.00000000000001421, 54.99999999999999289, -16.97055937655931501 ) ) ;
#4255=EDGE_LOOP ( 'NONE', ( #3628, #10111 ) ) ;
#4259=DIRECTION ( 'NONE',  ( 0.000000000000000000, 0.000000000000000000, 1.000000000000000000 ) ) ;
#4264=EDGE_LOOP ( 'NONE', ( #1722, #9044 ) ) ;
#4274=DIRECTION ( 'NONE',  ( 0.000000000000000000, 1.000000000000000000, 0.000000000000000000 ) ) ;
#4278=DIRECTION ( 'NONE',  ( -1.000000000000000000, -0.000000000000000000, -0.000000000000000000 ) ) ;
#4286=ORIENTED_EDGE ( 'NONE', *, *, #9599, .F. ) ;
#4302=DIRECTION ( 'NONE',  ( -1.000000000000000000, -0.000000000000000000, -0.000000000000000000 ) ) ;
#4310=ORIENTED_EDGE ( 'NONE', *, *, #4547, .F. ) ;
#4330=EDGE_CURVE ( 'NONE', #9331, #6771, #7509, .T. ) ;
#4331=AXIS2_PLACEMENT_3D ( 'NONE', #1878, #9192, #4645 ) ;
#4336=ORIENTED_EDGE ( 'NONE', *, *, #8896, .T. ) ;
#4340=EDGE_CURVE ( 'NONE', #4456, #6484, #7, .T. ) ;
#4342=FACE_OUTER_BOUND ( 'NONE', #10677, .T. ) ;
#4348=ORIENTED_EDGE ( 'NONE', *, *, #11280, .F. ) ;
#4360=DIRECTION ( 'NONE',  ( -1.000000000000000000, -0.000000000000000000, -0.000000000000000000 ) ) ;
#4364=ORIENTED_EDGE ( 'NONE', *, *, #3449, .T. ) ;
#4372=DIRECTION ( 'NONE',  ( 0.000000000000000000, 0.000000000000000000, 1.000000000000000000 ) ) ;
#4373=FACE_BOUND ( 'NONE', #4255, .T. ) ;
#4383=CARTESIAN_POINT ( 'NONE',  ( -78.00000000000001421, 67.72792206135787296, -12.72791868944004534 ) ) ;
#4386=VERTEX_POINT ( 'NONE', #10534 ) ;
#4392=DIRECTION ( 'NONE',  ( 0.000000000000000000, 0.000000000000000000, 1.000000000000000000 ) ) ;
#4399=DIRECTION ( 'NONE',  ( 0.000000000000000000, 1.000000000000000000, 0.000000000000000000 ) ) ;
#4403=VECTOR ( 'NONE', #3637, 1000.000000000000000 ) ;
#4405=CIRCLE ( 'NONE', #3826, 21.50000000000000000 ) ;
#4407=ORIENTED_EDGE ( 'NONE', *, *, #7782, .F. ) ;
#4414=ORIENTED_EDGE ( 'NONE', *, *, #8576, .T. ) ;
#4419=ADVANCED_FACE ( 'NONE', ( #9588 ), #2273, .F. ) ;
#4430=EDGE_LOOP ( 'NONE', ( #1513, #908 ) ) ;
#4432=DIRECTION ( 'NONE',  ( -1.000000000000000000, -0.000000000000000000, -0.000000000000000000 ) ) ;
#4443=DIRECTION ( 'NONE',  ( 0.000000000000000000, 1.000000000000000000, 0.000000000000000000 ) ) ;
#4449=ORIENTED_EDGE ( 'NONE', *, *, #11785, .F. ) ;
#4456=VERTEX_POINT ( 'NONE', #8923 ) ;
#4459=CARTESIAN_POINT ( 'NONE',  ( -80.00000000000001421, 67.72792206135787296, 2.742644059037073312 ) ) ;
#4474=( LENGTH_UNIT ( ) NAMED_UNIT ( * ) SI_UNIT ( .MILLI., .METRE. ) );
#4486=DIRECTION ( 'NONE',  ( 0.000000000000000000, 0.000000000000000000, 1.000000000000000000 ) ) ;
#4489=DIRECTION ( 'NONE',  ( 0.000000000000000000, 0.000000000000000000, -1.000000000000000000 ) ) ;
#4491=DIRECTION ( 'NONE',  ( -1.000000000000000000, -0.000000000000000000, -0.000000000000000000 ) ) ;
#4492=VERTEX_POINT ( 'NONE', #9095 ) ;
#4493=DIRECTION ( 'NONE',  ( -1.000000000000000000, -0.000000000000000000, -0.000000000000000000 ) ) ;
#4510=DIRECTION ( 'NONE',  ( 0.000000000000000000, 1.000000000000000000, 0.000000000000000000 ) ) ;
#4516=CIRCLE ( 'NONE', #6064, 1.500000000000001332 ) ;
#4524=CIRCLE ( 'NONE', #1546, 1.500000000000001332 ) ;
#4530=EDGE_LOOP ( 'NONE', ( #6309, #11675 ) ) ;
#4535=AXIS2_PLACEMENT_3D ( 'NONE', #1075, #2099, #3903 ) ;
#4539=AXIS2_PLACEMENT_3D ( 'NONE', #5131, #10501, #11454 ) ;
#4541=DIRECTION ( 'NONE',  ( 0.000000000000000000, 1.000000000000000000, 0.000000000000000000 ) ) ;
#4542=ORIENTED_EDGE ( 'NONE', *, *, #6385, .F. ) ;
#4547=EDGE_CURVE ( 'NONE', #6864, #8080, #9402, .T. ) ;
#4552=LINE ( 'NONE', #4728, #11431 ) ;
#4569=CARTESIAN_POINT ( 'NONE',  ( -78.00000000000000000, 55.00000000000000000, 0.000000000000000000 ) ) ;
#4570=EDGE_LOOP ( 'NONE', ( #11040, #8302, #1484, #8922 ) ) ;
#4572=CYLINDRICAL_SURFACE ( 'NONE', #4801, 1.499999999999999556 ) ;
#4576=DIRECTION ( 'NONE',  ( -1.000000000000000000, -0.000000000000000000, -0.000000000000000000 ) ) ;
#4578=VERTEX_POINT ( 'NONE', #3646 ) ;
#4582=VECTOR ( 'NONE', #11162, 1000.000000000000000 ) ;
#4593=FACE_OUTER_BOUND ( 'NONE', #3501, .T. ) ;
#4605=DIRECTION ( 'NONE',  ( -1.000000000000000000, -0.000000000000000000, -0.000000000000000000 ) ) ;
#4608=CIRCLE ( 'NONE', #965, 1.500000000000001332 ) ;
#4609=CARTESIAN_POINT ( 'NONE',  ( -80.00000000000001421, 54.99999999999998579, -6.985278002320760571 ) ) ;
#4619=EDGE_CURVE ( 'NONE', #1706, #11337, #7882, .T. ) ;
#4621=CYLINDRICAL_SURFACE ( 'NONE', #1474, 1.499999999999999556 ) ;
#4623=AXIS2_PLACEMENT_3D ( 'NONE', #9265, #5813, #2927 ) ;
#4635=EDGE_CURVE ( 'NONE', #2349, #11145, #5784, .T. ) ;
#4642=EDGE_LOOP ( 'NONE', ( #6275, #1003, #114, #770 ) ) ;
#4645=DIRECTION ( 'NONE',  ( 0.000000000000000000, 1.000000000000000000, 0.000000000000000000 ) ) ;
#4646=EDGE_LOOP ( 'NONE', ( #5603, #4105, #3176, #4859 ) ) ;
#4659=DIRECTION ( 'NONE',  ( 1.000000000000000000, 0.000000000000000000, 0.000000000000000000 ) ) ;
#4662=VERTEX_POINT ( 'NONE', #10823 ) ;
#4676=ADVANCED_FACE ( 'NONE', ( #3940 ), #2143, .F. ) ;
#4683=DIRECTION ( 'NONE',  ( 0.000000000000000000, 1.000000000000000000, 0.000000000000000000 ) ) ;
#4684=FACE_BOUND ( 'NONE', #11330, .T. ) ;
#4688=AXIS2_PLACEMENT_3D ( 'NONE', #3102, #4840, #2190 ) ;
#4696=ORIENTED_EDGE ( 'NONE', *, *, #11196, .F. ) ;
#4701=EDGE_CURVE ( 'NONE', #4778, #11556, #10358, .T. ) ;
#4706=ORIENTED_EDGE ( 'NONE', *, *, #8065, .F. ) ;
#4716=DIRECTION ( 'NONE',  ( -1.000000000000000000, -0.000000000000000000, -0.000000000000000000 ) ) ;
#4723=AXIS2_PLACEMENT_3D ( 'NONE', #650, #4491, #7200 ) ;
#4726=AXIS2_PLACEMENT_3D ( 'NONE', #9336, #1192, #2874 ) ;
#4728=CARTESIAN_POINT ( 'NONE',  ( -78.00000000000001421, 54.99999999999999289, -15.47055937655931501 ) ) ;
#4734=ORIENTED_EDGE ( 'NONE', *, *, #3812, .F. ) ;
#4738=AXIS2_PLACEMENT_3D ( 'NONE', #6164, #8011, #1383 ) ;
#4747=CARTESIAN_POINT ( 'NONE',  ( -80.00000000000001421, 59.24264068711927678, 4.242644059037073312 ) ) ;
#4750=FACE_BOUND ( 'NONE', #3380, .T. ) ;
#4752=VECTOR ( 'NONE', #9099, 1000.000000000000000 ) ;
#4753=CARTESIAN_POINT ( 'NONE',  ( -80.00000000000001421, 59.24264068711927678, 4.242644059037073312 ) ) ;
#4757=DIRECTION ( 'NONE',  ( -1.000000000000000000, -0.000000000000000000, -0.000000000000000000 ) ) ;
#4758=ORIENTED_EDGE ( 'NONE', *, *, #2480, .T. ) ;
#4772=CARTESIAN_POINT ( 'NONE',  ( -78.00000000000001421, 46.51471862576140381, -8.485278002320759683 ) ) ;
#4773=CARTESIAN_POINT ( 'NONE',  ( -80.00000000000002842, 42.27207793864211283, 12.72792543327562775 ) ) ;
#4778=VERTEX_POINT ( 'NONE', #10163 ) ;
#4784=AXIS2_PLACEMENT_3D ( 'NONE', #4383, #7029, #10772 ) ;
#4790=DIRECTION ( 'NONE',  ( 0.000000000000000000, 1.000000000000000000, 0.000000000000000000 ) ) ;
#4801=AXIS2_PLACEMENT_3D ( 'NONE', #119, #11807, #3671 ) ;
#4816=AXIS2_PLACEMENT_3D ( 'NONE', #1236, #3043, #7547 ) ;
#4817=DIRECTION ( 'NONE',  ( -1.000000000000000000, -0.000000000000000000, -0.000000000000000000 ) ) ;
#4818=VECTOR ( 'NONE', #6969, 1000.000000000000000 ) ;
#4819=EDGE_LOOP ( 'NONE', ( #9284, #7998 ) ) ;
#4822=DIRECTION ( 'NONE',  ( -1.000000000000000000, -0.000000000000000000, -0.000000000000000000 ) ) ;
#4823=ORIENTED_EDGE ( 'NONE', *, *, #1557, .T. ) ;
#4827=CIRCLE ( 'NONE', #9191, 1.500000000000001332 ) ;
#4829=DIRECTION ( 'NONE',  ( -1.000000000000000000, -0.000000000000000000, -0.000000000000000000 ) ) ;
#4832=FACE_OUTER_BOUND ( 'NONE', #3329, .T. ) ;
#4833=ADVANCED_FACE ( 'NONE', ( #9737 ), #513, .F. ) ;
#4835=DIRECTION ( 'NONE',  ( -1.000000000000000000, -0.000000000000000000, -0.000000000000000000 ) ) ;
#4839=CARTESIAN_POINT ( 'NONE',  ( -80.00000000000001421, 63.48528137423857487, -8.485278002320759683 ) ) ;
#4840=DIRECTION ( 'NONE',  ( -1.000000000000000000, -0.000000000000000000, -0.000000000000000000 ) ) ;
#4841=DIRECTION ( 'NONE',  ( -1.000000000000000000, -0.000000000000000000, -0.000000000000000000 ) ) ;
#4844=EDGE_LOOP ( 'NONE', ( #6921, #1400 ) ) ;
#4859=ORIENTED_EDGE ( 'NONE', *, *, #11249, .T. ) ;
#4861=FACE_BOUND ( 'NONE', #959, .T. ) ;
#4863=EDGE_CURVE ( 'NONE', #2849, #89, #10871, .T. ) ;
#4867=DIRECTION ( 'NONE',  ( 0.000000000000000000, 1.000000000000000000, 0.000000000000000000 ) ) ;
#4871=CARTESIAN_POINT ( 'NONE',  ( -78.00000000000002842, 38.02943725152282184, 1.500003371917797867 ) ) ;
#4872=AXIS2_PLACEMENT_3D ( 'NONE', #8860, #6231, #9691 ) ;
#4875=DIRECTION ( 'NONE',  ( -1.000000000000000000, -0.000000000000000000, -0.000000000000000000 ) ) ;
#4880=VERTEX_POINT ( 'NONE', #7836 ) ;
#4888=CARTESIAN_POINT ( 'NONE',  ( -78.00000000000002842, 38.02943725152282184, 3.371917797929946392E-06 ) ) ;
#4890=EDGE_CURVE ( 'NONE', #7763, #6131, #8215, .T. ) ;
#4906=AXIS2_PLACEMENT_3D ( 'NONE', #441, #8536, #2179 ) ;
#4907=CARTESIAN_POINT ( 'NONE',  ( -80.00000000000002842, 46.51471862576140381, 8.485284746156354529 ) ) ;
#4911=AXIS2_PLACEMENT_3D ( 'NONE', #3635, #2795, #8428 ) ;
#4914=DIRECTION ( 'NONE',  ( -1.000000000000000000, -0.000000000000000000, -0.000000000000000000 ) ) ;
#4915=DIRECTION ( 'NONE',  ( -1.000000000000000000, -0.000000000000000000, -0.000000000000000000 ) ) ;
#4918=VERTEX_POINT ( 'NONE', #3161 ) ;
#4923=CIRCLE ( 'NONE', #7794, 1.500000000000001332 ) ;
#4924=LINE ( 'NONE', #11370, #10834 ) ;
#4925=EDGE_CURVE ( 'NONE', #69, #1770, #5347, .T. ) ;
#4931=CIRCLE ( 'NONE', #6273, 1.500000000000001332 ) ;
#4938=CIRCLE ( 'NONE', #2823, 1.500000000000001332 ) ;
#4954=ORIENTED_EDGE ( 'NONE', *, *, #8773, .T. ) ;
#4958=FACE_OUTER_BOUND ( 'NONE', #348, .T. ) ;
#4959=UNCERTAINTY_MEASURE_WITH_UNIT (LENGTH_MEASURE( 1.000000000000000082E-05 ), #4474, 'distance_accuracy_value', 'NONE');
#4961=AXIS2_PLACEMENT_3D ( 'NONE', #2614, #1710, #6397 ) ;
#4971=ORIENTED_EDGE ( 'NONE', *, *, #11272, .T. ) ;
#4978=VERTEX_POINT ( 'NONE', #9914 ) ;
#4981=AXIS2_PLACEMENT_3D ( 'NONE', #11228, #4841, #10510 ) ;
#4986=DIRECTION ( 'NONE',  ( -1.000000000000000000, -0.000000000000000000, -0.000000000000000000 ) ) ;
#4988=AXIS2_PLACEMENT_3D ( 'NONE', #8978, #10936, #7188 ) ;
#4989=ORIENTED_EDGE ( 'NONE', *, *, #4330, .F. ) ;
#4993=ORIENTED_EDGE ( 'NONE', *, *, #11634, .F. ) ;
#4998=DIRECTION ( 'NONE',  ( -1.000000000000000000, -0.000000000000000000, -0.000000000000000000 ) ) ;
#5009=CARTESIAN_POINT ( 'NONE',  ( -78.00000000000002842, 46.51471862576140381, -1.499996628082201244 ) ) ;
#5010=DIRECTION ( 'NONE',  ( 0.000000000000000000, 1.000000000000000000, 0.000000000000000000 ) ) ;
#5015=ADVANCED_FACE ( 'NONE', ( #3459 ), #5488, .F. ) ;
#5016=ORIENTED_EDGE ( 'NONE', *, *, #9614, .T. ) ;
#5017=DIRECTION ( 'NONE',  ( -1.000000000000000000, -0.000000000000000000, -0.000000000000000000 ) ) ;
#5023=AXIS2_PLACEMENT_3D ( 'NONE', #3414, #7027, #5279 ) ;
#5033=ORIENTED_EDGE ( 'NONE', *, *, #5587, .F. ) ;
#5042=FACE_BOUND ( 'NONE', #11269, .T. ) ;
#5043=FACE_BOUND ( 'NONE', #10167, .T. ) ;
#5049=ORIENTED_EDGE ( 'NONE', *, *, #6777, .F. ) ;
#5050=CARTESIAN_POINT ( 'NONE',  ( -78.00000000000001421, 67.72792206135787296, 4.242644059037073312 ) ) ;
#5052=FACE_OUTER_BOUND ( 'NONE', #10072, .T. ) ;
#5055=EDGE_CURVE ( 'NONE', #2528, #9349, #8785, .T. ) ;
#5066=EDGE_CURVE ( 'NONE', #9906, #4880, #5733, .T. ) ;
#5068=DIRECTION ( 'NONE',  ( -1.000000000000000000, -0.000000000000000000, -0.000000000000000000 ) ) ;
#5070=DIRECTION ( 'NONE',  ( -1.000000000000000000, -0.000000000000000000, -0.000000000000000000 ) ) ;
#5075=EDGE_CURVE ( 'NONE', #3587, #10599, #10927, .T. ) ;
#5080=ADVANCED_FACE ( 'NONE', ( #5260 ), #1768, .F. ) ;
#5086=LINE ( 'NONE', #10574, #7800 ) ;
#5097=EDGE_LOOP ( 'NONE', ( #10727, #2495, #974, #11366 ) ) ;
#5108=DIRECTION ( 'NONE',  ( -1.000000000000000000, -0.000000000000000000, -0.000000000000000000 ) ) ;
#5110=FACE_OUTER_BOUND ( 'NONE', #10226, .T. ) ;
#5130=ORIENTED_EDGE ( 'NONE', *, *, #3370, .T. ) ;
#5131=CARTESIAN_POINT ( 'NONE',  ( -78.00000000000001421, 59.24264068711928388, -12.72791868944003824 ) ) ;
#5133=ORIENTED_EDGE ( 'NONE', *, *, #7055, .T. ) ;
#5137=ORIENTED_EDGE ( 'NONE', *, *, #6473, .T. ) ;
#5140=ADVANCED_FACE ( 'NONE', ( #920 ), #8127, .F. ) ;
#5146=DIRECTION ( 'NONE',  ( 0.000000000000000000, 1.000000000000000000, 0.000000000000000000 ) ) ;
#5160=DIRECTION ( 'NONE',  ( -1.000000000000000000, -0.000000000000000000, -0.000000000000000000 ) ) ;
#5164=CARTESIAN_POINT ( 'NONE',  ( -80.00000000000000000, 54.99999999999999289, 3.371917797062584654E-06 ) ) ;
#5168=ORIENTED_EDGE ( 'NONE', *, *, #3309, .T. ) ;
#5169=EDGE_CURVE ( 'NONE', #6748, #8286, #7840, .T. ) ;
#5174=CIRCLE ( 'NONE', #10693, 1.500000000000001332 ) ;
#5179=CARTESIAN_POINT ( 'NONE',  ( -78.00000000000001421, 67.72792206135787296, -2.742637315201482462 ) ) ;
#5181=DIRECTION ( 'NONE',  ( -1.000000000000000000, -0.000000000000000000, -0.000000000000000000 ) ) ;
#5188=CARTESIAN_POINT ( 'NONE',  ( -80.00000000000001421, 67.72792206135787296, 14.22792543327562775 ) ) ;
#5189=CIRCLE ( 'NONE', #3652, 1.500000000000001332 ) ;
#5197=ORIENTED_EDGE ( 'NONE', *, *, #3187, .F. ) ;
#5202=AXIS2_PLACEMENT_3D ( 'NONE', #34, #7199, #5505 ) ;
#5210=CARTESIAN_POINT ( 'NONE',  ( -78.00000000000002842, 38.02943725152282184, 1.500003371917797867 ) ) ;
#5216=FACE_BOUND ( 'NONE', #2102, .T. ) ;
#5220=ORIENTED_EDGE ( 'NONE', *, *, #9346, .F. ) ;
#5235=CARTESIAN_POINT ( 'NONE',  ( -80.00000000000002842, 38.02943725152282184, 1.500003371917797867 ) ) ;
#5239=VERTEX_POINT ( 'NONE', #5235 ) ;
#5248=CARTESIAN_POINT ( 'NONE',  ( -80.00000000000001421, 42.27207793864211283, -14.22791868944003646 ) ) ;
#5251=ORIENTED_EDGE ( 'NONE', *, *, #4162, .F. ) ;
#5259=EDGE_CURVE ( 'NONE', #10459, #3587, #2670, .T. ) ;
#5260=FACE_OUTER_BOUND ( 'NONE', #5282, .T. ) ;
#5267=CARTESIAN_POINT ( 'NONE',  ( -78.00000000000001421, 67.72792206135787296, 14.22792543327562775 ) ) ;
#5272=FACE_BOUND ( 'NONE', #10636, .T. ) ;
#5277=CARTESIAN_POINT ( 'NONE',  ( -80.00000000000001421, 59.24264068711928388, -14.22791868944003646 ) ) ;
#5279=DIRECTION ( 'NONE',  ( 0.000000000000000000, 1.000000000000000000, 0.000000000000000000 ) ) ;
#5281=CARTESIAN_POINT ( 'NONE',  ( -78.00000000000001421, 54.99999999999998579, -9.985278002320759683 ) ) ;
#5282=EDGE_LOOP ( 'NONE', ( #6834, #7893, #10443, #10371 ) ) ;
#5284=ORIENTED_EDGE ( 'NONE', *, *, #11785, .T. ) ;
#5287=DIRECTION ( 'NONE',  ( 0.000000000000000000, 1.000000000000000000, 0.000000000000000000 ) ) ;
#5290=CARTESIAN_POINT ( 'NONE',  ( -78.00000000000001421, 59.24264068711928388, -14.22791868944003646 ) ) ;
#5292=ORIENTED_EDGE ( 'NONE', *, *, #1076, .T. ) ;
#5294=DIRECTION ( 'NONE',  ( 0.000000000000000000, 0.000000000000000000, 1.000000000000000000 ) ) ;
#5297=EDGE_CURVE ( 'NONE', #642, #10867, #9494, .T. ) ;
#5302=LINE ( 'NONE', #8056, #5675 ) ;
#5312=ORIENTED_EDGE ( 'NONE', *, *, #6847, .F. ) ;
#5320=ORIENTED_EDGE ( 'NONE', *, *, #6841, .T. ) ;
#5326=CARTESIAN_POINT ( 'NONE',  ( -78.00000000000002842, 54.99999999999998579, 16.97056612039490986 ) ) ;
#5328=CYLINDRICAL_SURFACE ( 'NONE', #8440, 1.500000000000000000 ) ;
#5329=CARTESIAN_POINT ( 'NONE',  ( -78.00000000000001421, 59.24264068711928388, -12.72791868944003824 ) ) ;
#5343=EDGE_LOOP ( 'NONE', ( #8868, #6022, #9585, #3657 ) ) ;
#5347=CIRCLE ( 'NONE', #917, 1.500000000000001332 ) ;
#5352=VECTOR ( 'NONE', #753, 1000.000000000000000 ) ;
#5353=DIRECTION ( 'NONE',  ( -1.000000000000000000, -0.000000000000000000, -0.000000000000000000 ) ) ;
#5360=AXIS2_PLACEMENT_3D ( 'NONE', #9259, #10034, #929 ) ;
#5363=VERTEX_POINT ( 'NONE', #5651 ) ;
#5369=EDGE_LOOP ( 'NONE', ( #3956, #9098, #3145, #2155 ) ) ;
#5375=AXIS2_PLACEMENT_3D ( 'NONE', #3018, #9299, #6686 ) ;
#5376=CARTESIAN_POINT ( 'NONE',  ( -78.00000000000000000, 55.00000000000000000, 0.000000000000000000 ) ) ;
#5382=CIRCLE ( 'NONE', #3848, 1.500000000000001332 ) ;
#5389=FACE_OUTER_BOUND ( 'NONE', #2733, .T. ) ;
#5391=ORIENTED_EDGE ( 'NONE', *, *, #3187, .T. ) ;
#5393=DIRECTION ( 'NONE',  ( 0.000000000000000000, 1.000000000000000000, 0.000000000000000000 ) ) ;
#5400=CIRCLE ( 'NONE', #14, 1.500000000000001332 ) ;
#5415=DIRECTION ( 'NONE',  ( 0.000000000000000000, 1.000000000000000000, 0.000000000000000000 ) ) ;
#5419=DIRECTION ( 'NONE',  ( 0.000000000000000000, 1.000000000000000000, 0.000000000000000000 ) ) ;
#5423=VERTEX_POINT ( 'NONE', #9236 ) ;
#5426=ADVANCED_FACE ( 'NONE', ( #10469 ), #2954, .F. ) ;
#5430=EDGE_LOOP ( 'NONE', ( #11846, #1590, #1250, #3005 ) ) ;
#5432=ADVANCED_FACE ( 'NONE', ( #9639, #5598, #528, #7517, #7851, #4684, #10246, #9584, #1380, #8336, #11480, #11422, #11138, #245, #3291, #3786, #7455, #1984, #3909, #2044, #2893, #5717, #8689, #6562, #1142, #1085, #4750, #6845, #5042, #471 ), #4128, .T. ) ;
#5442=CYLINDRICAL_SURFACE ( 'NONE', #1714, 1.499999999999999556 ) ;
#5443=ORIENTED_EDGE ( 'NONE', *, *, #72, .F. ) ;
#5447=VERTEX_POINT ( 'NONE', #2451 ) ;
#5451=CARTESIAN_POINT ( 'NONE',  ( -78.00000000000002842, 50.75735931288069480, 2.742644059037076865 ) ) ;
#5452=DIRECTION ( 'NONE',  ( -1.000000000000000000, -0.000000000000000000, -0.000000000000000000 ) ) ;
#5465=DIRECTION ( 'NONE',  ( -1.000000000000000000, -0.000000000000000000, -0.000000000000000000 ) ) ;
#5466=ORIENTED_EDGE ( 'NONE', *, *, #8705, .F. ) ;
#5470=FACE_OUTER_BOUND ( 'NONE', #9660, .T. ) ;
#5476=CIRCLE ( 'NONE', #3752, 1.500000000000001332 ) ;
#5477=CARTESIAN_POINT ( 'NONE',  ( -78.00000000000002842, 50.75735931288069480, 5.742644059037076865 ) ) ;
#5488=CYLINDRICAL_SURFACE ( 'NONE', #9154, 1.500000000000000444 ) ;
#5491=ORIENTED_EDGE ( 'NONE', *, *, #2710, .T. ) ;
#5505=DIRECTION ( 'NONE',  ( 0.000000000000000000, 1.000000000000000000, 0.000000000000000000 ) ) ;
#5508=ADVANCED_FACE ( 'NONE', ( #6117 ), #10818, .F. ) ;
#5509=ORIENTED_EDGE ( 'NONE', *, *, #2138, .T. ) ;
#5516=VERTEX_POINT ( 'NONE', #7911 ) ;
#5522=CARTESIAN_POINT ( 'NONE',  ( -78.00000000000001421, 42.27207793864211283, -12.72791868944003824 ) ) ;
#5527=AXIS2_PLACEMENT_3D ( 'NONE', #688, #4360, #8012 ) ;
#5528=ADVANCED_FACE ( 'NONE', ( #5389 ), #11775, .F. ) ;
#5529=DIRECTION ( 'NONE',  ( -1.000000000000000000, -0.000000000000000000, -0.000000000000000000 ) ) ;
#5535=AXIS2_PLACEMENT_3D ( 'NONE', #5376, #7242, #10865 ) ;
#5538=ORIENTED_EDGE ( 'NONE', *, *, #3463, .T. ) ;
#5543=AXIS2_PLACEMENT_3D ( 'NONE', #3656, #7438, #3597 ) ;
#5545=ADVANCED_FACE ( 'NONE', ( #3523 ), #11540, .F. ) ;
#5549=ORIENTED_EDGE ( 'NONE', *, *, #1030, .T. ) ;
#5554=ORIENTED_EDGE ( 'NONE', *, *, #9679, .F. ) ;
#5568=ORIENTED_EDGE ( 'NONE', *, *, #10188, .T. ) ;
#5572=DIRECTION ( 'NONE',  ( -1.000000000000000000, -0.000000000000000000, -0.000000000000000000 ) ) ;
#5579=EDGE_CURVE ( 'NONE', #4918, #642, #10314, .T. ) ;
#5582=ORIENTED_EDGE ( 'NONE', *, *, #2710, .F. ) ;
#5587=EDGE_CURVE ( 'NONE', #8286, #6748, #1889, .T. ) ;
#5588=CYLINDRICAL_SURFACE ( 'NONE', #9901, 1.500000000000000444 ) ;
#5592=EDGE_CURVE ( 'NONE', #43, #9873, #4204, .T. ) ;
#5598=FACE_BOUND ( 'NONE', #4430, .T. ) ;
#5603=ORIENTED_EDGE ( 'NONE', *, *, #6691, .F. ) ;
#5613=EDGE_LOOP ( 'NONE', ( #3304, #128 ) ) ;
#5614=DIRECTION ( 'NONE',  ( 0.000000000000000000, 0.000000000000000000, 1.000000000000000000 ) ) ;
#5621=DIRECTION ( 'NONE',  ( -1.000000000000000000, -0.000000000000000000, -0.000000000000000000 ) ) ;
#5624=ORIENTED_EDGE ( 'NONE', *, *, #1294, .T. ) ;
#5625=LINE ( 'NONE', #90, #590 ) ;
#5631=ORIENTED_EDGE ( 'NONE', *, *, #6188, .F. ) ;
#5635=CARTESIAN_POINT ( 'NONE',  ( -80.00000000000002842, 46.51471862576140381, 3.371917798797308130E-06 ) ) ;
#5636=DIRECTION ( 'NONE',  ( 0.000000000000000000, 0.000000000000000000, 1.000000000000000000 ) ) ;
#5641=VERTEX_POINT ( 'NONE', #8137 ) ;
#5642=DIRECTION ( 'NONE',  ( -1.000000000000000000, -0.000000000000000000, -0.000000000000000000 ) ) ;
#5646=CYLINDRICAL_SURFACE ( 'NONE', #6869, 1.499999999999999556 ) ;
#5651=CARTESIAN_POINT ( 'NONE',  ( -78.00000000000002842, 54.99999999999998579, 15.47056612039490986 ) ) ;
#5666=CARTESIAN_POINT ( 'NONE',  ( -80.00000000000002842, 38.02943725152282184, 3.371917797929946392E-06 ) ) ;
#5675=VECTOR ( 'NONE', #11700, 1000.000000000000000 ) ;
#5681=MECHANICAL_DESIGN_GEOMETRIC_PRESENTATION_REPRESENTATION('',(#7397),#9110);
#5685=EDGE_CURVE ( 'NONE', #8040, #7395, #11837, .T. ) ;
#5697=CARTESIAN_POINT ( 'NONE',  ( -78.00000000000001421, 63.48528137423857487, -8.485278002320759683 ) ) ;
#5704=EDGE_LOOP ( 'NONE', ( #749, #411, #8667, #5915 ) ) ;
#5706=CIRCLE ( 'NONE', #6472, 1.500000000000001332 ) ;
#5717=FACE_BOUND ( 'NONE', #6170, .T. ) ;
#5733=CIRCLE ( 'NONE', #1120, 1.500000000000001332 ) ;
#5743=CARTESIAN_POINT ( 'NONE',  ( -78.00000000000002842, 42.27207793864211283, 4.242644059037075976 ) ) ;
#5744=CIRCLE ( 'NONE', #1137, 1.500000000000001332 ) ;
#5745=ADVANCED_FACE ( 'NONE', ( #9500 ), #269, .F. ) ;
#5747=CARTESIAN_POINT ( 'NONE',  ( -78.00000000000002842, 42.27207793864211283, 14.22792543327562775 ) ) ;
#5760=DIRECTION ( 'NONE',  ( -1.000000000000000000, -0.000000000000000000, -0.000000000000000000 ) ) ;
#5763=ORIENTED_EDGE ( 'NONE', *, *, #11646, .F. ) ;
#5765=FACE_BOUND ( 'NONE', #635, .T. ) ;
#5770=CARTESIAN_POINT ( 'NONE',  ( -78.00000000000001421, 67.72792206135787296, -2.742637315201482462 ) ) ;
#5776=DIRECTION ( 'NONE',  ( 0.000000000000000000, 1.000000000000000000, 0.000000000000000000 ) ) ;
#5779=EDGE_LOOP ( 'NONE', ( #8863, #3238, #3032, #9369 ) ) ;
#5780=EDGE_CURVE ( 'NONE', #7355, #10318, #5744, .T. ) ;
#5784=CIRCLE ( 'NONE', #3099, 1.500000000000001332 ) ;
#5785=DIRECTION ( 'NONE',  ( 0.000000000000000000, 1.000000000000000000, 0.000000000000000000 ) ) ;
#5789=LINE ( 'NONE', #10968, #11091 ) ;
#5806=CARTESIAN_POINT ( 'NONE',  ( -80.00000000000002842, 50.75735931288069480, 4.242644059037076865 ) ) ;
#5807=CARTESIAN_POINT ( 'NONE',  ( -80.00000000000001421, 63.48528137423857487, 6.985284746156351865 ) ) ;
#5813=DIRECTION ( 'NONE',  ( -1.000000000000000000, -0.000000000000000000, -0.000000000000000000 ) ) ;
#5820=EDGE_CURVE ( 'NONE', #6131, #7763, #5174, .T. ) ;
#5849=DIRECTION ( 'NONE',  ( -1.000000000000000000, -0.000000000000000000, -0.000000000000000000 ) ) ;
#5852=VERTEX_POINT ( 'NONE', #3035 ) ;
#5867=FACE_OUTER_BOUND ( 'NONE', #8315, .T. ) ;
#5871=EDGE_LOOP ( 'NONE', ( #622, #666 ) ) ;
#5876=CARTESIAN_POINT ( 'NONE',  ( -78.00000000000001421, 50.75735931288069480, -14.22791868944003646 ) ) ;
#5879=ORIENTED_EDGE ( 'NONE', *, *, #11280, .T. ) ;
#5881=FACE_BOUND ( 'NONE', #3929, .T. ) ;
#5884=AXIS2_PLACEMENT_3D ( 'NONE', #7493, #4605, #2865 ) ;
#5889=ORIENTED_EDGE ( 'NONE', *, *, #7423, .F. ) ;
#5899=CARTESIAN_POINT ( 'NONE',  ( -80.00000000000001421, 63.48528137423857487, 8.485284746156350977 ) ) ;
#5900=EDGE_LOOP ( 'NONE', ( #9837, #2204, #3455, #8371 ) ) ;
#5906=VECTOR ( 'NONE', #2523, 1000.000000000000000 ) ;
#5915=ORIENTED_EDGE ( 'NONE', *, *, #1152, .T. ) ;
#5920=UNCERTAINTY_MEASURE_WITH_UNIT (LENGTH_MEASURE( 1.000000000000000082E-05 ), #6512, 'distance_accuracy_value', 'NONE');
#5939=DIRECTION ( 'NONE',  ( 0.000000000000000000, 1.000000000000000000, 0.000000000000000000 ) ) ;
#5941=EDGE_LOOP ( 'NONE', ( #2530, #1841, #5292, #252 ) ) ;
#5955=CARTESIAN_POINT ( 'NONE',  ( -78.00000000000002842, 50.75735931288069480, 12.72792543327563131 ) ) ;
#5956=EDGE_CURVE ( 'NONE', #5423, #1264, #3141, .T. ) ;
#5967=CARTESIAN_POINT ( 'NONE',  ( -80.00000000000001421, 50.75735931288069480, -4.242637315201482906 ) ) ;
#5973=EDGE_LOOP ( 'NONE', ( #6509, #862, #10132, #3846 ) ) ;
#5978=CIRCLE ( 'NONE', #11298, 1.500000000000001332 ) ;
#5982=DIRECTION ( 'NONE',  ( -1.000000000000000000, -0.000000000000000000, -0.000000000000000000 ) ) ;
#5987=CIRCLE ( 'NONE', #5023, 1.500000000000001332 ) ;
#5992=CYLINDRICAL_SURFACE ( 'NONE', #4130, 1.499999999999999556 ) ;
#5999=DIRECTION ( 'NONE',  ( -1.000000000000000000, -0.000000000000000000, -0.000000000000000000 ) ) ;
#6001=ADVANCED_FACE ( 'NONE', ( #5052 ), #183, .F. ) ;
#6004=VERTEX_POINT ( 'NONE', #3008 ) ;
#6006=DIRECTION ( 'NONE',  ( 0.000000000000000000, 0.000000000000000000, 1.000000000000000000 ) ) ;
#6009=DIRECTION ( 'NONE',  ( 0.000000000000000000, 0.000000000000000000, 1.000000000000000000 ) ) ;
#6010=DIRECTION ( 'NONE',  ( -1.000000000000000000, -0.000000000000000000, -0.000000000000000000 ) ) ;
#6014=CARTESIAN_POINT ( 'NONE',  ( -80.00000000000002842, 46.51471862576140381, 9.985284746156354529 ) ) ;
#6022=ORIENTED_EDGE ( 'NONE', *, *, #4863, .F. ) ;
#6026=AXIS2_PLACEMENT_3D ( 'NONE', #9386, #1180, #1307 ) ;
#6028=ADVANCED_FACE ( 'NONE', ( #5110 ), #600, .F. ) ;
#6034=ORIENTED_EDGE ( 'NONE', *, *, #8066, .F. ) ;
#6035=CARTESIAN_POINT ( 'NONE',  ( -80.00000000000001421, 59.24264068711927678, -5.742637315201482906 ) ) ;
#6036=EDGE_CURVE ( 'NONE', #9669, #5516, #7471, .T. ) ;
#6038=VERTEX_POINT ( 'NONE', #7802 ) ;
#6046=CARTESIAN_POINT ( 'NONE',  ( -80.00000000000002842, 46.51471862576140381, -1.499996628082201244 ) ) ;
#6050=DIRECTION ( 'NONE',  ( 0.000000000000000000, 1.000000000000000000, 0.000000000000000000 ) ) ;
#6063=CARTESIAN_POINT ( 'NONE',  ( -80.00000000000000000, 55.00000000000000000, 0.000000000000000000 ) ) ;
#6064=AXIS2_PLACEMENT_3D ( 'NONE', #1158, #4829, #1278 ) ;
#6068=CARTESIAN_POINT ( 'NONE',  ( -78.00000000000001421, 46.51471862576140381, -6.985278002320760571 ) ) ;
#6072=DIRECTION ( 'NONE',  ( 1.000000000000000000, 0.000000000000000000, 0.000000000000000000 ) ) ;
#6074=EDGE_CURVE ( 'NONE', #7355, #4880, #8933, .T. ) ;
#6075=AXIS2_PLACEMENT_3D ( 'NONE', #5967, #9604, #1396 ) ;
#6079=DIRECTION ( 'NONE',  ( -1.000000000000000000, -0.000000000000000000, -0.000000000000000000 ) ) ;
#6082=CARTESIAN_POINT ( 'NONE',  ( -80.00000000000001421, 67.72792206135787296, -4.242637315201482906 ) ) ;
#6091=DIRECTION ( 'NONE',  ( -1.000000000000000000, -0.000000000000000000, -0.000000000000000000 ) ) ;
#6095=ORIENTED_EDGE ( 'NONE', *, *, #8065, .T. ) ;
#6099=EDGE_CURVE ( 'NONE', #8080, #6864, #4405, .T. ) ;
#6112=DIRECTION ( 'NONE',  ( 0.000000000000000000, 0.000000000000000000, 1.000000000000000000 ) ) ;
#6115=EDGE_LOOP ( 'NONE', ( #4026, #11004 ) ) ;
#6117=FACE_OUTER_BOUND ( 'NONE', #4101, .T. ) ;
#6118=CARTESIAN_POINT ( 'NONE',  ( -78.00000000000001421, 54.99999999999999289, -15.47055937655931501 ) ) ;
#6121=ORIENTED_EDGE ( 'NONE', *, *, #2288, .F. ) ;
#6128=CIRCLE ( 'NONE', #8414, 1.500000000000001332 ) ;
#6130=CARTESIAN_POINT ( 'NONE',  ( -80.00000000000000000, 55.00000000000000000, 0.000000000000000000 ) ) ;
#6131=VERTEX_POINT ( 'NONE', #2399 ) ;
#6135=DIRECTION ( 'NONE',  ( 0.000000000000000000, 1.000000000000000000, 0.000000000000000000 ) ) ;
#6136=DIRECTION ( 'NONE',  ( 0.000000000000000000, 1.000000000000000000, 0.000000000000000000 ) ) ;
#6139=DIRECTION ( 'NONE',  ( -1.000000000000000000, -0.000000000000000000, -0.000000000000000000 ) ) ;
#6141=ORIENTED_EDGE ( 'NONE', *, *, #9822, .F. ) ;
#6144=DIRECTION ( 'NONE',  ( 0.000000000000000000, 1.000000000000000000, 0.000000000000000000 ) ) ;
#6146=DIRECTION ( 'NONE',  ( 0.000000000000000000, 0.000000000000000000, 1.000000000000000000 ) ) ;
#6150=ORIENTED_EDGE ( 'NONE', *, *, #956, .F. ) ;
#6151=DIRECTION ( 'NONE',  ( -1.000000000000000000, -0.000000000000000000, -0.000000000000000000 ) ) ;
#6159=AXIS2_PLACEMENT_3D ( 'NONE', #424, #11376, #3009 ) ;
#6164=CARTESIAN_POINT ( 'NONE',  ( 0.000000000000000000, 0.000000000000000000, 0.000000000000000000 ) ) ;
#6167=DIRECTION ( 'NONE',  ( -1.000000000000000000, -0.000000000000000000, -0.000000000000000000 ) ) ;
#6170=EDGE_LOOP ( 'NONE', ( #2294, #5320 ) ) ;
#6177=EDGE_CURVE ( 'NONE', #7683, #7763, #4203, .T. ) ;
#6188=EDGE_CURVE ( 'NONE', #9256, #2813, #3250, .T. ) ;
#6191=LINE ( 'NONE', #1389, #4818 ) ;
#6194=VERTEX_POINT ( 'NONE', #7977 ) ;
#6195=DIRECTION ( 'NONE',  ( 0.000000000000000000, 0.000000000000000000, 1.000000000000000000 ) ) ;
#6196=ORIENTED_EDGE ( 'NONE', *, *, #4635, .F. ) ;
#6200=DIRECTION ( 'NONE',  ( 0.000000000000000000, 1.000000000000000000, 0.000000000000000000 ) ) ;
#6202=ORIENTED_EDGE ( 'NONE', *, *, #5579, .F. ) ;
#6203=DIRECTION ( 'NONE',  ( -1.000000000000000000, -0.000000000000000000, -0.000000000000000000 ) ) ;
#6205=CARTESIAN_POINT ( 'NONE',  ( -78.00000000000001421, 46.51471862576140381, -9.985278002320759683 ) ) ;
#6208=FACE_OUTER_BOUND ( 'NONE', #5369, .T. ) ;
#6219=DIRECTION ( 'NONE',  ( -1.000000000000000000, -0.000000000000000000, -0.000000000000000000 ) ) ;
#6222=ORIENTED_EDGE ( 'NONE', *, *, #5685, .T. ) ;
#6224=ADVANCED_FACE ( 'NONE', ( #11614 ), #10714, .F. ) ;
#6231=DIRECTION ( 'NONE',  ( -1.000000000000000000, -0.000000000000000000, -0.000000000000000000 ) ) ;
#6232=DIRECTION ( 'NONE',  ( -1.000000000000000000, -0.000000000000000000, -0.000000000000000000 ) ) ;
#6241=VERTEX_POINT ( 'NONE', #5281 ) ;
#6245=ORIENTED_EDGE ( 'NONE', *, *, #11646, .T. ) ;
#6247=CIRCLE ( 'NONE', #10901, 1.500000000000001332 ) ;
#6263=EDGE_CURVE ( 'NONE', #10429, #5239, #7663, .T. ) ;
#6270=VECTOR ( 'NONE', #2160, 1000.000000000000000 ) ;
#6271=EDGE_LOOP ( 'NONE', ( #6968, #5391, #631, #8483 ) ) ;
#6272=DIRECTION ( 'NONE',  ( -1.000000000000000000, -0.000000000000000000, -0.000000000000000000 ) ) ;
#6273=AXIS2_PLACEMENT_3D ( 'NONE', #2637, #709, #4443 ) ;
#6275=ORIENTED_EDGE ( 'NONE', *, *, #11517, .F. ) ;
#6278=AXIS2_PLACEMENT_3D ( 'NONE', #250, #6625, #10253 ) ;
#6291=CARTESIAN_POINT ( 'NONE',  ( -78.00000000000002842, 54.99999999999998579, 8.485284746156354529 ) ) ;
#6293=EDGE_CURVE ( 'NONE', #1850, #11230, #4019, .T. ) ;
#6294=CARTESIAN_POINT ( 'NONE',  ( -78.00000000000001421, 71.97056274847716395, 1.500003371917795425 ) ) ;
#6297=CIRCLE ( 'NONE', #11021, 1.500000000000001332 ) ;
#6298=ORIENTED_EDGE ( 'NONE', *, *, #6099, .F. ) ;
#6300=FACE_OUTER_BOUND ( 'NONE', #10187, .T. ) ;
#6307=ORIENTED_EDGE ( 'NONE', *, *, #6830, .T. ) ;
#6309=ORIENTED_EDGE ( 'NONE', *, *, #6385, .T. ) ;
#6318=AXIS2_PLACEMENT_3D ( 'NONE', #1494, #1661, #7015 ) ;
#6322=CARTESIAN_POINT ( 'NONE',  ( -80.00000000000000000, 54.99999999999999289, 3.371917797062584654E-06 ) ) ;
#6341=AXIS2_PLACEMENT_3D ( 'NONE', #7591, #4835, #7534 ) ;
#6349=CARTESIAN_POINT ( 'NONE',  ( -78.00000000000002842, 42.27207793864211283, 12.72792543327562775 ) ) ;
#6350=CARTESIAN_POINT ( 'NONE',  ( -78.00000000000000000, 54.99999999999999289, -1.499996628082203021 ) ) ;
#6367=AXIS2_PLACEMENT_3D ( 'NONE', #669, #727, #4399 ) ;
#6377=ORIENTED_EDGE ( 'NONE', *, *, #7055, .F. ) ;
#6378=LINE ( 'NONE', #2537, #10798 ) ;
#6385=EDGE_CURVE ( 'NONE', #1831, #5363, #8995, .T. ) ;
#6394=( NAMED_UNIT ( * ) PLANE_ANGLE_UNIT ( ) SI_UNIT ( $, .RADIAN. ) );
#6395=ADVANCED_FACE ( 'NONE', ( #10035 ), #5442, .F. ) ;
#6397=DIRECTION ( 'NONE',  ( 0.000000000000000000, 1.000000000000000000, 0.000000000000000000 ) ) ;
#6405=ORIENTED_EDGE ( 'NONE', *, *, #5820, .T. ) ;
#6432=DIRECTION ( 'NONE',  ( -1.000000000000000000, -0.000000000000000000, -0.000000000000000000 ) ) ;
#6436=CIRCLE ( 'NONE', #4331, 1.500000000000001332 ) ;
#6438=ORIENTED_EDGE ( 'NONE', *, *, #3551, .T. ) ;
#6439=VECTOR ( 'NONE', #248, 1000.000000000000000 ) ;
#6440=ADVANCED_FACE ( 'NONE', ( #3580 ), #2685, .F. ) ;
#6442=ORIENTED_EDGE ( 'NONE', *, *, #7630, .F. ) ;
#6446=ORIENTED_EDGE ( 'NONE', *, *, #2574, .F. ) ;
#6459=AXIS2_PLACEMENT_3D ( 'NONE', #7838, #11467, #3109 ) ;
#6464=CARTESIAN_POINT ( 'NONE',  ( -78.00000000000002842, 42.27207793864211283, 12.72792543327562775 ) ) ;
#6465=ORIENTED_EDGE ( 'NONE', *, *, #2183, .F. ) ;
#6470=ADVANCED_FACE ( 'NONE', ( #2799 ), #7250, .F. ) ;
#6472=AXIS2_PLACEMENT_3D ( 'NONE', #4102, #5982, #6991 ) ;
#6473=EDGE_CURVE ( 'NONE', #9349, #2528, #10126, .T. ) ;
#6476=CARTESIAN_POINT ( 'NONE',  ( -78.00000000000000000, 54.99999999999999289, 3.371917797062584654E-06 ) ) ;
#6482=EDGE_LOOP ( 'NONE', ( #8136, #2153 ) ) ;
#6484=VERTEX_POINT ( 'NONE', #930 ) ;
#6491=CARTESIAN_POINT ( 'NONE',  ( -78.00000000000001421, 54.99999999999998579, -6.985278002320760571 ) ) ;
#6494=CARTESIAN_POINT ( 'NONE',  ( -78.00000000000001421, 50.75735931288069480, -4.242637315201482906 ) ) ;
#6496=PRODUCT_CONTEXT ( 'NONE', #2098, 'mechanical' ) ;
#6498=CARTESIAN_POINT ( 'NONE',  ( -78.00000000000001421, 50.75735931288069480, -5.742637315201482906 ) ) ;
#6500=ORIENTED_EDGE ( 'NONE', *, *, #9822, .T. ) ;
#6504=EDGE_CURVE ( 'NONE', #5852, #7713, #88, .T. ) ;
#6507=CIRCLE ( 'NONE', #4981, 1.500000000000001332 ) ;
#6509=ORIENTED_EDGE ( 'NONE', *, *, #3645, .F. ) ;
#6512=( LENGTH_UNIT ( ) NAMED_UNIT ( * ) SI_UNIT ( .MILLI., .METRE. ) );
#6518=AXIS2_PLACEMENT_3D ( 'NONE', #6291, #9923, #1830 ) ;
#6519=VERTEX_POINT ( 'NONE', #10756 ) ;
#6522=FACE_OUTER_BOUND ( 'NONE', #9943, .T. ) ;
#6530=CIRCLE ( 'NONE', #2690, 1.500000000000001332 ) ;
#6556=DIRECTION ( 'NONE',  ( -1.000000000000000000, -0.000000000000000000, -0.000000000000000000 ) ) ;
#6561=CARTESIAN_POINT ( 'NONE',  ( -78.00000000000001421, 63.48528137423857487, -8.485278002320759683 ) ) ;
#6562=FACE_BOUND ( 'NONE', #9132, .T. ) ;
#6567=EDGE_LOOP ( 'NONE', ( #3181, #2227, #2801, #7102 ) ) ;
#6569=LINE ( 'NONE', #7343, #3456 ) ;
#6571=ADVANCED_FACE ( 'NONE', ( #10217 ), #150, .F. ) ;
#6581=ORIENTED_EDGE ( 'NONE', *, *, #9679, .T. ) ;
#6584=CYLINDRICAL_SURFACE ( 'NONE', #6643, 1.499999999999999556 ) ;
#6589=ORIENTED_EDGE ( 'NONE', *, *, #11249, .F. ) ;
#6599=AXIS2_PLACEMENT_3D ( 'NONE', #6349, #5621, #27 ) ;
#6600=DIRECTION ( 'NONE',  ( 0.000000000000000000, 0.000000000000000000, 1.000000000000000000 ) ) ;
#6613=DIRECTION ( 'NONE',  ( -1.000000000000000000, -0.000000000000000000, -0.000000000000000000 ) ) ;
#6614=VERTEX_POINT ( 'NONE', #5747 ) ;
#6620=CIRCLE ( 'NONE', #7003, 1.500000000000001332 ) ;
#6622=CARTESIAN_POINT ( 'NONE',  ( -78.00000000000001421, 59.24264068711927678, -5.742637315201482906 ) ) ;
#6625=DIRECTION ( 'NONE',  ( -1.000000000000000000, -0.000000000000000000, -0.000000000000000000 ) ) ;
#6630=CIRCLE ( 'NONE', #9104, 1.500000000000001332 ) ;
#6637=CIRCLE ( 'NONE', #11777, 1.500000000000001332 ) ;
#6643=AXIS2_PLACEMENT_3D ( 'NONE', #4772, #7538, #7304 ) ;
#6648=CARTESIAN_POINT ( 'NONE',  ( -78.00000000000002842, 50.75735931288069480, 11.22792543327563131 ) ) ;
#6654=EDGE_LOOP ( 'NONE', ( #5284, #6438 ) ) ;
#6656=CARTESIAN_POINT ( 'NONE',  ( -80.00000000000000000, 54.99999999999999289, -1.499996628082203021 ) ) ;
#6675=VECTOR ( 'NONE', #5465, 1000.000000000000000 ) ;
#6676=ORIENTED_EDGE ( 'NONE', *, *, #5956, .T. ) ;
#6686=DIRECTION ( 'NONE',  ( 0.000000000000000000, 0.000000000000000000, 1.000000000000000000 ) ) ;
#6691=EDGE_CURVE ( 'NONE', #10318, #9906, #2856, .T. ) ;
#6695=DIRECTION ( 'NONE',  ( -1.000000000000000000, -0.000000000000000000, -0.000000000000000000 ) ) ;
#6705=DIRECTION ( 'NONE',  ( -1.000000000000000000, -0.000000000000000000, -0.000000000000000000 ) ) ;
#6708=DIRECTION ( 'NONE',  ( -1.000000000000000000, -0.000000000000000000, -0.000000000000000000 ) ) ;
#6713=CARTESIAN_POINT ( 'NONE',  ( -78.00000000000001421, 50.75735931288069480, -2.742637315201482462 ) ) ;
#6714=VECTOR ( 'NONE', #3197, 1000.000000000000000 ) ;
#6720=LINE ( 'NONE', #2149, #3332 ) ;
#6728=FACE_BOUND ( 'NONE', #2400, .T. ) ;
#6746=DIRECTION ( 'NONE',  ( 0.000000000000000000, 1.000000000000000000, 0.000000000000000000 ) ) ;
#6748=VERTEX_POINT ( 'NONE', #3371 ) ;
#6760=EDGE_CURVE ( 'NONE', #89, #2384, #3318, .T. ) ;
#6766=CARTESIAN_POINT ( 'NONE',  ( -78.00000000000002842, 59.24264068711927678, 12.72792543327563131 ) ) ;
#6767=LINE ( 'NONE', #1229, #3351 ) ;
#6771=VERTEX_POINT ( 'NONE', #4459 ) ;
#6777=EDGE_CURVE ( 'NONE', #9231, #1770, #10607, .T. ) ;
#6779=DIRECTION ( 'NONE',  ( -1.000000000000000000, -0.000000000000000000, -0.000000000000000000 ) ) ;
#6792=CYLINDRICAL_SURFACE ( 'NONE', #9140, 21.50000000000000000 ) ;
#6800=DIRECTION ( 'NONE',  ( 0.000000000000000000, 1.000000000000000000, 0.000000000000000000 ) ) ;
#6802=FACE_OUTER_BOUND ( 'NONE', #6271, .T. ) ;
#6804=EDGE_LOOP ( 'NONE', ( #8234, #5549 ) ) ;
#6808=CARTESIAN_POINT ( 'NONE',  ( -80.00000000000001421, 63.48528137423857487, -9.985278002320759683 ) ) ;
#6811=CARTESIAN_POINT ( 'NONE',  ( -78.00000000000001421, 63.48528137423857487, 9.985284746156350977 ) ) ;
#6813=LINE ( 'NONE', #2423, #1293 ) ;
#6818=ORIENTED_EDGE ( 'NONE', *, *, #5169, .T. ) ;
#6823=DIRECTION ( 'NONE',  ( 0.000000000000000000, 1.000000000000000000, 0.000000000000000000 ) ) ;
#6826=DIRECTION ( 'NONE',  ( 0.000000000000000000, 1.000000000000000000, 0.000000000000000000 ) ) ;
#6827=EDGE_CURVE ( 'NONE', #241, #7948, #3675, .T. ) ;
#6828=CARTESIAN_POINT ( 'NONE',  ( -80.00000000000001421, 67.72792206135787296, -4.242637315201482906 ) ) ;
#6830=EDGE_CURVE ( 'NONE', #9231, #10654, #4827, .T. ) ;
#6834=ORIENTED_EDGE ( 'NONE', *, *, #9295, .F. ) ;
#6841=EDGE_CURVE ( 'NONE', #10318, #7355, #3261, .T. ) ;
#6845=FACE_BOUND ( 'NONE', #2505, .T. ) ;
#6847=EDGE_CURVE ( 'NONE', #11145, #7332, #9897, .T. ) ;
#6860=ORIENTED_EDGE ( 'NONE', *, *, #382, .T. ) ;
#6864=VERTEX_POINT ( 'NONE', #9007 ) ;
#6869=AXIS2_PLACEMENT_3D ( 'NONE', #1977, #6556, #9348 ) ;
#6870=DIRECTION ( 'NONE',  ( 0.000000000000000000, 1.000000000000000000, 0.000000000000000000 ) ) ;
#6876=ORIENTED_EDGE ( 'NONE', *, *, #5259, .T. ) ;
#6880=CARTESIAN_POINT ( 'NONE',  ( -80.00000000000001421, 59.24264068711928388, -11.22791868944003824 ) ) ;
#6881=AXIS2_PLACEMENT_3D ( 'NONE', #11586, #10573, #4115 ) ;
#6887=LINE ( 'NONE', #10515, #9318 ) ;
#6892=CARTESIAN_POINT ( 'NONE',  ( -78.00000000000002842, 54.99999999999998579, 8.485284746156354529 ) ) ;
#6900=AXIS2_PLACEMENT_3D ( 'NONE', #8551, #7657, #332 ) ;
#6906=EDGE_CURVE ( 'NONE', #10565, #1970, #3552, .T. ) ;
#6907=CARTESIAN_POINT ( 'NONE',  ( -78.00000000000000000, 55.00000000000000000, 0.000000000000000000 ) ) ;
#6911=DIRECTION ( 'NONE',  ( -1.000000000000000000, -0.000000000000000000, -0.000000000000000000 ) ) ;
#6913=CIRCLE ( 'NONE', #8821, 1.500000000000001332 ) ;
#6915=EDGE_CURVE ( 'NONE', #2813, #9256, #4038, .T. ) ;
#6921=ORIENTED_EDGE ( 'NONE', *, *, #1181, .F. ) ;
#6934=CYLINDRICAL_SURFACE ( 'NONE', #517, 1.500000000000000000 ) ;
#6937=ORIENTED_EDGE ( 'NONE', *, *, #11634, .T. ) ;
#6940=VECTOR ( 'NONE', #4098, 1000.000000000000000 ) ;
#6944=ORIENTED_EDGE ( 'NONE', *, *, #11357, .F. ) ;
#6946=CARTESIAN_POINT ( 'NONE',  ( -80.00000000000001421, 54.99999999999998579, -8.485278002320759683 ) ) ;
#6947=DIRECTION ( 'NONE',  ( 0.000000000000000000, 1.000000000000000000, 0.000000000000000000 ) ) ;
#6948=DIRECTION ( 'NONE',  ( -1.000000000000000000, -0.000000000000000000, -0.000000000000000000 ) ) ;
#6950=ORIENTED_EDGE ( 'NONE', *, *, #6691, .T. ) ;
#6956=DIRECTION ( 'NONE',  ( 0.000000000000000000, 1.000000000000000000, 0.000000000000000000 ) ) ;
#6959=EDGE_CURVE ( 'NONE', #2643, #8769, #6913, .T. ) ;
#6966=ADVANCED_FACE ( 'NONE', ( #10064 ), #10908, .F. ) ;
#6968=ORIENTED_EDGE ( 'NONE', *, *, #2201, .F. ) ;
#6969=DIRECTION ( 'NONE',  ( -1.000000000000000000, -0.000000000000000000, -0.000000000000000000 ) ) ;
#6972=ORIENTED_EDGE ( 'NONE', *, *, #960, .T. ) ;
#6979=ADVANCED_FACE ( 'NONE', ( #5470 ), #4572, .F. ) ;
#6983=CIRCLE ( 'NONE', #6026, 1.500000000000001332 ) ;
#6985=CARTESIAN_POINT ( 'NONE',  ( -78.00000000000002842, 54.99999999999998579, 6.985284746156355418 ) ) ;
#6988=DIRECTION ( 'NONE',  ( -1.000000000000000000, -0.000000000000000000, -0.000000000000000000 ) ) ;
#6991=DIRECTION ( 'NONE',  ( 0.000000000000000000, 1.000000000000000000, 0.000000000000000000 ) ) ;
#7000=CARTESIAN_POINT ( 'NONE',  ( -80.00000000000001421, 42.27207793864211283, -12.72791868944003824 ) ) ;
#7003=AXIS2_PLACEMENT_3D ( 'NONE', #7160, #11690, #3212 ) ;
#7015=DIRECTION ( 'NONE',  ( 0.000000000000000000, 0.000000000000000000, -1.000000000000000000 ) ) ;
#7019=EDGE_LOOP ( 'NONE', ( #10570, #9497, #11244, #1330 ) ) ;
#7024=CARTESIAN_POINT ( 'NONE',  ( -80.00000000000001421, 59.24264068711928388, -12.72791868944003824 ) ) ;
#7026=CIRCLE ( 'NONE', #10058, 1.500000000000001332 ) ;
#7027=DIRECTION ( 'NONE',  ( -1.000000000000000000, -0.000000000000000000, -0.000000000000000000 ) ) ;
#7029=DIRECTION ( 'NONE',  ( -1.000000000000000000, -0.000000000000000000, -0.000000000000000000 ) ) ;
#7030=ORIENTED_EDGE ( 'NONE', *, *, #10177, .T. ) ;
#7032=CYLINDRICAL_SURFACE ( 'NONE', #11297, 1.500000000000000444 ) ;
#7037=DIRECTION ( 'NONE',  ( -1.000000000000000000, -0.000000000000000000, -0.000000000000000000 ) ) ;
#7044=CIRCLE ( 'NONE', #4726, 1.500000000000001332 ) ;
#7050=AXIS2_PLACEMENT_3D ( 'NONE', #4569, #8160, #4392 ) ;
#7055=EDGE_CURVE ( 'NONE', #11654, #6519, #3465, .T. ) ;
#7056=DIRECTION ( 'NONE',  ( 0.000000000000000000, 1.000000000000000000, 0.000000000000000000 ) ) ;
#7065=EDGE_CURVE ( 'NONE', #10744, #5423, #2507, .T. ) ;
#7071=CARTESIAN_POINT ( 'NONE',  ( -78.00000000000002842, 54.99999999999998579, 9.985284746156354529 ) ) ;
#7078=DIRECTION ( 'NONE',  ( 0.000000000000000000, 1.000000000000000000, 0.000000000000000000 ) ) ;
#7079=FACE_BOUND ( 'NONE', #4036, .T. ) ;
#7084=AXIS2_PLACEMENT_3D ( 'NONE', #1724, #700, #4486 ) ;
#7091=CARTESIAN_POINT ( 'NONE',  ( -78.00000000000001421, 63.48528137423857487, 1.500003371917795425 ) ) ;
#7102=ORIENTED_EDGE ( 'NONE', *, *, #3891, .T. ) ;
#7104=CARTESIAN_POINT ( 'NONE',  ( -80.00000000000001421, 63.48528137423857487, -8.485278002320759683 ) ) ;
#7105=CIRCLE ( 'NONE', #8060, 1.500000000000001332 ) ;
#7106=ADVANCED_FACE ( 'NONE', ( #7388 ), #11015, .F. ) ;
#7110=AXIS2_PLACEMENT_3D ( 'NONE', #7454, #2827, #10123 ) ;
#7114=DIRECTION ( 'NONE',  ( -1.000000000000000000, -0.000000000000000000, -0.000000000000000000 ) ) ;
#7132=CARTESIAN_POINT ( 'NONE',  ( -78.00000000000001421, 54.99999999999999289, -16.97055937655931501 ) ) ;
#7135=CARTESIAN_POINT ( 'NONE',  ( -78.00000000000001421, 67.72792206135787296, 5.742644059037073312 ) ) ;
#7139=FACE_BOUND ( 'NONE', #1702, .T. ) ;
#7157=CARTESIAN_POINT ( 'NONE',  ( -78.00000000000001421, 54.99999999999998579, -8.485278002320759683 ) ) ;
#7160=CARTESIAN_POINT ( 'NONE',  ( -78.00000000000001421, 42.27207793864211283, -12.72791868944003824 ) ) ;
#7162=CARTESIAN_POINT ( 'NONE',  ( -78.00000000000001421, 67.72792206135787296, -4.242637315201482906 ) ) ;
#7168=DIRECTION ( 'NONE',  ( 0.000000000000000000, 1.000000000000000000, 0.000000000000000000 ) ) ;
#7176=DIRECTION ( 'NONE',  ( -1.000000000000000000, -0.000000000000000000, -0.000000000000000000 ) ) ;
#7183=ORIENTED_EDGE ( 'NONE', *, *, #9645, .T. ) ;
#7188=DIRECTION ( 'NONE',  ( 0.000000000000000000, 0.000000000000000000, 1.000000000000000000 ) ) ;
#7191=DIRECTION ( 'NONE',  ( 0.000000000000000000, 1.000000000000000000, 0.000000000000000000 ) ) ;
#7192=FACE_BOUND ( 'NONE', #583, .T. ) ;
#7195=ADVANCED_FACE ( 'NONE', ( #10308 ), #9597, .F. ) ;
#7198=EDGE_LOOP ( 'NONE', ( #4310, #6298 ) ) ;
#7199=DIRECTION ( 'NONE',  ( -1.000000000000000000, -0.000000000000000000, -0.000000000000000000 ) ) ;
#7200=DIRECTION ( 'NONE',  ( 0.000000000000000000, 0.000000000000000000, 1.000000000000000000 ) ) ;
#7201=ORIENTED_EDGE ( 'NONE', *, *, #1731, .T. ) ;
#7202=FACE_OUTER_BOUND ( 'NONE', #4646, .T. ) ;
#7208=AXIS2_PLACEMENT_3D ( 'NONE', #2508, #8912, #5146 ) ;
#7209=EDGE_LOOP ( 'NONE', ( #5197, #3698, #5538, #4336 ) ) ;
#7210=EDGE_CURVE ( 'NONE', #518, #5239, #244, .T. ) ;
#7216=DIRECTION ( 'NONE',  ( -1.000000000000000000, -0.000000000000000000, -0.000000000000000000 ) ) ;
#7217=LINE ( 'NONE', #11684, #6675 ) ;
#7220=CIRCLE ( 'NONE', #2032, 1.500000000000001332 ) ;
#7221=CYLINDRICAL_SURFACE ( 'NONE', #1441, 1.499999999999999556 ) ;
#7223=CARTESIAN_POINT ( 'NONE',  ( -78.00000000000002842, 42.27207793864211283, 11.22792543327562775 ) ) ;
#7231=AXIS2_PLACEMENT_3D ( 'NONE', #1102, #11338, #5614 ) ;
#7236=AXIS2_PLACEMENT_3D ( 'NONE', #2375, #9510, #6050 ) ;
#7242=DIRECTION ( 'NONE',  ( 1.000000000000000000, 0.000000000000000000, 0.000000000000000000 ) ) ;
#7244=CIRCLE ( 'NONE', #2059, 1.500000000000001332 ) ;
#7249=CARTESIAN_POINT ( 'NONE',  ( -78.00000000000002842, 42.27207793864211283, 5.742644059037075088 ) ) ;
#7250=CYLINDRICAL_SURFACE ( 'NONE', #6518, 1.499999999999999556 ) ;
#7258=ORIENTED_EDGE ( 'NONE', *, *, #9059, .T. ) ;
#7271=CARTESIAN_POINT ( 'NONE',  ( -78.00000000000001421, 67.72792206135787296, -12.72791868944004534 ) ) ;
#7273=AXIS2_PLACEMENT_3D ( 'NONE', #10047, #11843, #8386 ) ;
#7279=DIRECTION ( 'NONE',  ( -1.000000000000000000, -0.000000000000000000, -0.000000000000000000 ) ) ;
#7282=VECTOR ( 'NONE', #10595, 1000.000000000000000 ) ;
#7285=EDGE_LOOP ( 'NONE', ( #1162, #9316, #7615, #3091 ) ) ;
#7286=CARTESIAN_POINT ( 'NONE',  ( -78.00000000000000000, 55.00000000000000000, 21.50000000000000000 ) ) ;
#7287=ORIENTED_EDGE ( 'NONE', *, *, #10188, .F. ) ;
#7289=AXIS2_PLACEMENT_3D ( 'NONE', #2296, #2409, #8768 ) ;
#7291=EDGE_LOOP ( 'NONE', ( #3558, #8379 ) ) ;
#7294=AXIS2_PLACEMENT_3D ( 'NONE', #7104, #1516, #6144 ) ;
#7296=ORIENTED_EDGE ( 'NONE', *, *, #11176, .T. ) ;
#7300=EDGE_LOOP ( 'NONE', ( #11002, #7505, #1128, #10376 ) ) ;
#7304=DIRECTION ( 'NONE',  ( 0.000000000000000000, 0.000000000000000000, 1.000000000000000000 ) ) ;
#7314=ADVANCED_FACE ( 'NONE', ( #771 ), #7032, .F. ) ;
#7316=ORIENTED_EDGE ( 'NONE', *, *, #1692, .T. ) ;
#7318=FACE_OUTER_BOUND ( 'NONE', #7368, .T. ) ;
#7321=AXIS2_PLACEMENT_3D ( 'NONE', #2772, #5529, #4683 ) ;
#7322=DIRECTION ( 'NONE',  ( -1.000000000000000000, -0.000000000000000000, -0.000000000000000000 ) ) ;
#7332=VERTEX_POINT ( 'NONE', #9651 ) ;
#7333=CARTESIAN_POINT ( 'NONE',  ( -78.00000000000002842, 50.75735931288069480, 4.242644059037076865 ) ) ;
#7343=CARTESIAN_POINT ( 'NONE',  ( -78.00000000000002842, 54.99999999999998579, 18.47056612039490986 ) ) ;
#7355=VERTEX_POINT ( 'NONE', #11617 ) ;
#7367=DIRECTION ( 'NONE',  ( -1.000000000000000000, -0.000000000000000000, -0.000000000000000000 ) ) ;
#7368=EDGE_LOOP ( 'NONE', ( #7733, #4449, #9724, #3055 ) ) ;
#7370=CARTESIAN_POINT ( 'NONE',  ( -80.00000000000002842, 42.27207793864211283, 11.22792543327562775 ) ) ;
#7385=EDGE_LOOP ( 'NONE', ( #1203, #7599, #1448, #7582 ) ) ;
#7388=FACE_OUTER_BOUND ( 'NONE', #7385, .T. ) ;
#7392=CIRCLE ( 'NONE', #2222, 1.500000000000001332 ) ;
#7395=VERTEX_POINT ( 'NONE', #3419 ) ;
#7397=STYLED_ITEM('',(#11902),#8587);
#7407=SURFACE_STYLE_FILL_AREA ( #2674 ) ;
#7409=ORIENTED_EDGE ( 'NONE', *, *, #9746, .F. ) ;
#7419=CIRCLE ( 'NONE', #11797, 1.500000000000001332 ) ;
#7420=FACE_OUTER_BOUND ( 'NONE', #11284, .T. ) ;
#7421=ADVANCED_FACE ( 'NONE', ( #2348 ), #540, .F. ) ;
#7423=EDGE_CURVE ( 'NONE', #322, #7683, #2120, .T. ) ;
#7429=CIRCLE ( 'NONE', #10471, 1.500000000000001332 ) ;
#7430=CARTESIAN_POINT ( 'NONE',  ( -78.00000000000001421, 42.27207793864211283, -14.22791868944003646 ) ) ;
#7433=DIRECTION ( 'NONE',  ( 0.000000000000000000, 1.000000000000000000, 0.000000000000000000 ) ) ;
#7438=DIRECTION ( 'NONE',  ( -1.000000000000000000, -0.000000000000000000, -0.000000000000000000 ) ) ;
#7440=ORIENTED_EDGE ( 'NONE', *, *, #10300, .F. ) ;
#7442=ORIENTED_EDGE ( 'NONE', *, *, #11853, .F. ) ;
#7454=CARTESIAN_POINT ( 'NONE',  ( -78.00000000000002842, 42.27207793864211283, 4.242644059037075976 ) ) ;
#7455=FACE_BOUND ( 'NONE', #7697, .T. ) ;
#7471=CIRCLE ( 'NONE', #2494, 1.500000000000001332 ) ;
#7472=FACE_OUTER_BOUND ( 'NONE', #79, .T. ) ;
#7480=ORIENTED_EDGE ( 'NONE', *, *, #1294, .F. ) ;
#7484=DIRECTION ( 'NONE',  ( 0.000000000000000000, 1.000000000000000000, 0.000000000000000000 ) ) ;
#7493=CARTESIAN_POINT ( 'NONE',  ( -80.00000000000002842, 59.24264068711927678, 12.72792543327563131 ) ) ;
#7505=ORIENTED_EDGE ( 'NONE', *, *, #72, .T. ) ;
#7507=ADVANCED_FACE ( 'NONE', ( #9808 ), #5328, .F. ) ;
#7509=LINE ( 'NONE', #10238, #780 ) ;
#7517=FACE_BOUND ( 'NONE', #2193, .T. ) ;
#7524=ORIENTED_EDGE ( 'NONE', *, *, #5297, .F. ) ;
#7534=DIRECTION ( 'NONE',  ( 0.000000000000000000, 1.000000000000000000, 0.000000000000000000 ) ) ;
#7538=DIRECTION ( 'NONE',  ( -1.000000000000000000, -0.000000000000000000, -0.000000000000000000 ) ) ;
#7540=FACE_OUTER_BOUND ( 'NONE', #2899, .T. ) ;
#7545=DIRECTION ( 'NONE',  ( 0.000000000000000000, 0.000000000000000000, 1.000000000000000000 ) ) ;
#7547=DIRECTION ( 'NONE',  ( 0.000000000000000000, 1.000000000000000000, 0.000000000000000000 ) ) ;
#7552=AXIS2_PLACEMENT_3D ( 'NONE', #8565, #2207, #1243 ) ;
#7565=DIRECTION ( 'NONE',  ( -1.000000000000000000, -0.000000000000000000, -0.000000000000000000 ) ) ;
#7575=PRODUCT_DEFINITION_FORMATION_WITH_SPECIFIED_SOURCE ( 'ANY', '', #2038, .NOT_KNOWN. ) ;
#7576=AXIS2_PLACEMENT_3D ( 'NONE', #4773, #9440, #3995 ) ;
#7580=CARTESIAN_POINT ( 'NONE',  ( -78.00000000000001421, 63.48528137423857487, 8.485284746156350977 ) ) ;
#7581=CARTESIAN_POINT ( 'NONE',  ( -78.00000000000001421, 46.51471862576140381, -8.485278002320759683 ) ) ;
#7582=ORIENTED_EDGE ( 'NONE', *, *, #1525, .F. ) ;
#7589=CYLINDRICAL_SURFACE ( 'NONE', #8750, 1.500000000000000000 ) ;
#7591=CARTESIAN_POINT ( 'NONE',  ( -80.00000000000002842, 50.75735931288069480, 12.72792543327563131 ) ) ;
#7599=ORIENTED_EDGE ( 'NONE', *, *, #956, .T. ) ;
#7604=CIRCLE ( 'NONE', #506, 1.500000000000001332 ) ;
#7605=DIRECTION ( 'NONE',  ( -1.000000000000000000, -0.000000000000000000, -0.000000000000000000 ) ) ;
#7607=CIRCLE ( 'NONE', #1475, 1.500000000000001332 ) ;
#7615=ORIENTED_EDGE ( 'NONE', *, *, #7825, .T. ) ;
#7618=FACE_BOUND ( 'NONE', #6115, .T. ) ;
#7629=EDGE_LOOP ( 'NONE', ( #10367, #341 ) ) ;
#7630=EDGE_CURVE ( 'NONE', #5363, #3229, #5625, .T. ) ;
#7655=DIRECTION ( 'NONE',  ( 0.000000000000000000, 0.000000000000000000, 1.000000000000000000 ) ) ;
#7657=DIRECTION ( 'NONE',  ( -1.000000000000000000, -0.000000000000000000, -0.000000000000000000 ) ) ;
#7663=CIRCLE ( 'NONE', #2485, 1.500000000000001332 ) ;
#7668=CYLINDRICAL_SURFACE ( 'NONE', #9770, 1.499999999999999556 ) ;
#7675=FACE_BOUND ( 'NONE', #2916, .T. ) ;
#7681=AXIS2_PLACEMENT_3D ( 'NONE', #10290, #11120, #8503 ) ;
#7682=FACE_OUTER_BOUND ( 'NONE', #8116, .T. ) ;
#7683=VERTEX_POINT ( 'NONE', #6294 ) ;
#7687=ORIENTED_EDGE ( 'NONE', *, *, #8705, .T. ) ;
#7691=AXIS2_PLACEMENT_3D ( 'NONE', #8093, #4659, #4489 ) ;
#7693=CIRCLE ( 'NONE', #3866, 1.500000000000001332 ) ;
#7697=EDGE_LOOP ( 'NONE', ( #5879, #2114 ) ) ;
#7707=CARTESIAN_POINT ( 'NONE',  ( -78.00000000000001421, 50.75735931288069480, -14.22791868944003646 ) ) ;
#7713=VERTEX_POINT ( 'NONE', #1762 ) ;
#7716=DIRECTION ( 'NONE',  ( 0.000000000000000000, 0.000000000000000000, 1.000000000000000000 ) ) ;
#7717=CARTESIAN_POINT ( 'NONE',  ( -78.00000000000002842, 46.51471862576140381, -1.499996628082201244 ) ) ;
#7723=DIRECTION ( 'NONE',  ( -1.000000000000000000, -0.000000000000000000, -0.000000000000000000 ) ) ;
#7724=DIRECTION ( 'NONE',  ( 0.000000000000000000, 1.000000000000000000, 0.000000000000000000 ) ) ;
#7733=ORIENTED_EDGE ( 'NONE', *, *, #8135, .F. ) ;
#7735=CARTESIAN_POINT ( 'NONE',  ( -80.00000000000002842, 50.75735931288069480, 2.742644059037076865 ) ) ;
#7755=AXIS2_PLACEMENT_3D ( 'NONE', #5743, #3878, #7655 ) ;
#7759=ORIENTED_EDGE ( 'NONE', *, *, #10730, .F. ) ;
#7761=CYLINDRICAL_SURFACE ( 'NONE', #1666, 1.499999999999999556 ) ;
#7763=VERTEX_POINT ( 'NONE', #3920 ) ;
#7767=CARTESIAN_POINT ( 'NONE',  ( -80.00000000000002842, 50.75735931288069480, 14.22792543327563131 ) ) ;
#7782=EDGE_CURVE ( 'NONE', #8790, #3229, #9593, .T. ) ;
#7790=DIRECTION ( 'NONE',  ( -1.000000000000000000, -0.000000000000000000, -0.000000000000000000 ) ) ;
#7794=AXIS2_PLACEMENT_3D ( 'NONE', #9056, #2648, #1622 ) ;
#7796=CARTESIAN_POINT ( 'NONE',  ( -78.00000000000002842, 54.99999999999998579, 16.97056612039490986 ) ) ;
#7800=VECTOR ( 'NONE', #11299, 1000.000000000000000 ) ;
#7802=CARTESIAN_POINT ( 'NONE',  ( -78.00000000000002842, 38.02943725152282184, -1.499996628082202133 ) ) ;
#7816=DIRECTION ( 'NONE',  ( -1.000000000000000000, -0.000000000000000000, -0.000000000000000000 ) ) ;
#7822=DIRECTION ( 'NONE',  ( 0.000000000000000000, 0.000000000000000000, 1.000000000000000000 ) ) ;
#7825=EDGE_CURVE ( 'NONE', #723, #4662, #3855, .T. ) ;
#7836=CARTESIAN_POINT ( 'NONE',  ( -80.00000000000001421, 63.48528137423857487, 1.500003371917795425 ) ) ;
#7838=CARTESIAN_POINT ( 'NONE',  ( -80.00000000000001421, 50.75735931288069480, -12.72791868944003824 ) ) ;
#7840=CIRCLE ( 'NONE', #5535, 21.50000000000000000 ) ;
#7851=FACE_BOUND ( 'NONE', #3471, .T. ) ;
#7862=CARTESIAN_POINT ( 'NONE',  ( -78.00000000000001421, 71.97056274847716395, 1.500003371917795425 ) ) ;
#7865=AXIS2_PLACEMENT_3D ( 'NONE', #9323, #10558, #11446 ) ;
#7866=PRODUCT_DEFINITION_CONTEXT ( 'detailed design', #2255, 'design' ) ;
#7872=ORIENTED_EDGE ( 'NONE', *, *, #2288, .T. ) ;
#7873=DIRECTION ( 'NONE',  ( 0.000000000000000000, 1.000000000000000000, 0.000000000000000000 ) ) ;
#7877=ORIENTED_EDGE ( 'NONE', *, *, #1332, .T. ) ;
#7882=CIRCLE ( 'NONE', #5202, 1.500000000000001332 ) ;
#7893=ORIENTED_EDGE ( 'NONE', *, *, #7630, .T. ) ;
#7911=CARTESIAN_POINT ( 'NONE',  ( -80.00000000000001421, 50.75735931288069480, -5.742637315201482906 ) ) ;
#7912=FACE_BOUND ( 'NONE', #479, .T. ) ;
#7929=CARTESIAN_POINT ( 'NONE',  ( -78.00000000000001421, 59.24264068711927678, 4.242644059037073312 ) ) ;
#7935=ADVANCED_FACE ( 'NONE', ( #7472 ), #10203, .F. ) ;
#7939=CARTESIAN_POINT ( 'NONE',  ( -80.00000000000001421, 54.99999999999999289, -16.97055937655931501 ) ) ;
#7940=ORIENTED_EDGE ( 'NONE', *, *, #4701, .T. ) ;
#7948=VERTEX_POINT ( 'NONE', #6808 ) ;
#7958=DIRECTION ( 'NONE',  ( -1.000000000000000000, -0.000000000000000000, -0.000000000000000000 ) ) ;
#7964=DIRECTION ( 'NONE',  ( -1.000000000000000000, -0.000000000000000000, -0.000000000000000000 ) ) ;
#7965=FACE_BOUND ( 'NONE', #4844, .T. ) ;
#7968=ORIENTED_EDGE ( 'NONE', *, *, #382, .F. ) ;
#7974=DIRECTION ( 'NONE',  ( -1.000000000000000000, -0.000000000000000000, -0.000000000000000000 ) ) ;
#7977=CARTESIAN_POINT ( 'NONE',  ( -78.00000000000000000, 54.99999999999999289, 1.500003371917797201 ) ) ;
#7992=CYLINDRICAL_SURFACE ( 'NONE', #10734, 1.499999999999999556 ) ;
#7994=AXIS2_PLACEMENT_3D ( 'NONE', #7157, #721, #6200 ) ;
#7998=ORIENTED_EDGE ( 'NONE', *, *, #11517, .T. ) ;
#8001=CARTESIAN_POINT ( 'NONE',  ( -80.00000000000001421, 67.72792206135787296, -12.72791868944004534 ) ) ;
#8006=VECTOR ( 'NONE', #6613, 1000.000000000000000 ) ;
#8007=VERTEX_POINT ( 'NONE', #11570 ) ;
#8008=EDGE_CURVE ( 'NONE', #8906, #2384, #7693, .T. ) ;
#8011=DIRECTION ( 'NONE',  ( 0.000000000000000000, 0.000000000000000000, 1.000000000000000000 ) ) ;
#8012=DIRECTION ( 'NONE',  ( 0.000000000000000000, 0.000000000000000000, 1.000000000000000000 ) ) ;
#8022=ORIENTED_EDGE ( 'NONE', *, *, #10655, .F. ) ;
#8025=CARTESIAN_POINT ( 'NONE',  ( -78.00000000000001421, 50.75735931288069480, -5.742637315201482906 ) ) ;
#8027=VECTOR ( 'NONE', #4302, 1000.000000000000000 ) ;
#8034=AXIS2_PLACEMENT_3D ( 'NONE', #3935, #6708, #6823 ) ;
#8039=CARTESIAN_POINT ( 'NONE',  ( -78.00000000000001421, 54.99999999999998579, -8.485278002320759683 ) ) ;
#8040=VERTEX_POINT ( 'NONE', #1403 ) ;
#8044=FACE_OUTER_BOUND ( 'NONE', #2998, .T. ) ;
#8045=DIRECTION ( 'NONE',  ( -1.000000000000000000, -0.000000000000000000, -0.000000000000000000 ) ) ;
#8051=DIRECTION ( 'NONE',  ( -1.000000000000000000, -0.000000000000000000, -0.000000000000000000 ) ) ;
#8056=CARTESIAN_POINT ( 'NONE',  ( -78.00000000000001421, 63.48528137423857487, -6.985278002320760571 ) ) ;
#8060=AXIS2_PLACEMENT_3D ( 'NONE', #9890, #11625, #4274 ) ;
#8062=EDGE_LOOP ( 'NONE', ( #10972, #11022 ) ) ;
#8065=EDGE_CURVE ( 'NONE', #3965, #7948, #8659, .T. ) ;
#8066=EDGE_CURVE ( 'NONE', #89, #2849, #5400, .T. ) ;
#8068=AXIS2_PLACEMENT_3D ( 'NONE', #2964, #1277, #8602 ) ;
#8080=VERTEX_POINT ( 'NONE', #2481 ) ;
#8089=DIRECTION ( 'NONE',  ( 0.000000000000000000, 0.000000000000000000, 1.000000000000000000 ) ) ;
#8090=FACE_BOUND ( 'NONE', #8539, .T. ) ;
#8093=CARTESIAN_POINT ( 'NONE',  ( -80.00000000000000000, 55.00000000000000000, 0.000000000000000000 ) ) ;
#8095=ORIENTED_EDGE ( 'NONE', *, *, #2500, .T. ) ;
#8106=DIRECTION ( 'NONE',  ( 0.000000000000000000, 1.000000000000000000, 0.000000000000000000 ) ) ;
#8107=CARTESIAN_POINT ( 'NONE',  ( -78.00000000000001421, 63.48528137423857487, -1.499996628082204797 ) ) ;
#8116=EDGE_LOOP ( 'NONE', ( #5033, #7877, #1257, #6465 ) ) ;
#8117=DIRECTION ( 'NONE',  ( 0.000000000000000000, 1.000000000000000000, 0.000000000000000000 ) ) ;
#8119=DIRECTION ( 'NONE',  ( 0.000000000000000000, 1.000000000000000000, 0.000000000000000000 ) ) ;
#8127=CYLINDRICAL_SURFACE ( 'NONE', #5527, 1.500000000000000000 ) ;
#8129=ORIENTED_EDGE ( 'NONE', *, *, #8476, .T. ) ;
#8135=EDGE_CURVE ( 'NONE', #849, #3307, #1345, .T. ) ;
#8136=ORIENTED_EDGE ( 'NONE', *, *, #587, .T. ) ;
#8137=CARTESIAN_POINT ( 'NONE',  ( -78.00000000000001421, 59.24264068711927678, -2.742637315201482462 ) ) ;
#8160=DIRECTION ( 'NONE',  ( -1.000000000000000000, -0.000000000000000000, -0.000000000000000000 ) ) ;
#8162=AXIS2_PLACEMENT_3D ( 'NONE', #369, #2406, #9773 ) ;
#8171=AXIS2_PLACEMENT_3D ( 'NONE', #7271, #10722, #8106 ) ;
#8173=AXIS2_PLACEMENT_3D ( 'NONE', #11240, #1244, #3950 ) ;
#8179=CIRCLE ( 'NONE', #2630, 1.500000000000001332 ) ;
#8189=EDGE_LOOP ( 'NONE', ( #4954, #6222 ) ) ;
#8194=LINE ( 'NONE', #7249, #2862 ) ;
#8210=ORIENTED_EDGE ( 'NONE', *, *, #9645, .F. ) ;
#8215=CIRCLE ( 'NONE', #6881, 1.500000000000001332 ) ;
#8232=ORIENTED_EDGE ( 'NONE', *, *, #6915, .T. ) ;
#8233=CARTESIAN_POINT ( 'NONE',  ( -78.00000000000001421, 42.27207793864211283, -14.22791868944003646 ) ) ;
#8234=ORIENTED_EDGE ( 'NONE', *, *, #3378, .T. ) ;
#8238=ORIENTED_EDGE ( 'NONE', *, *, #8684, .F. ) ;
#8241=AXIS2_PLACEMENT_3D ( 'NONE', #6322, #1751, #5415 ) ;
#8244=DIRECTION ( 'NONE',  ( -1.000000000000000000, -0.000000000000000000, -0.000000000000000000 ) ) ;
#8252=DIRECTION ( 'NONE',  ( -1.000000000000000000, -0.000000000000000000, -0.000000000000000000 ) ) ;
#8261=CARTESIAN_POINT ( 'NONE',  ( -80.00000000000002842, 50.75735931288069480, 12.72792543327563131 ) ) ;
#8262=ORIENTED_EDGE ( 'NONE', *, *, #3103, .T. ) ;
#8269=ORIENTED_EDGE ( 'NONE', *, *, #6263, .F. ) ;
#8271=ORIENTED_EDGE ( 'NONE', *, *, #8368, .F. ) ;
#8277=ORIENTED_EDGE ( 'NONE', *, *, #11026, .F. ) ;
#8280=DIRECTION ( 'NONE',  ( 0.000000000000000000, 1.000000000000000000, 0.000000000000000000 ) ) ;
#8285=DIRECTION ( 'NONE',  ( 0.000000000000000000, 1.000000000000000000, 0.000000000000000000 ) ) ;
#8286=VERTEX_POINT ( 'NONE', #2881 ) ;
#8288=ADVANCED_FACE ( 'NONE', ( #4342 ), #7992, .F. ) ;
#8290=EDGE_CURVE ( 'NONE', #11481, #2610, #5987, .T. ) ;
#8302=ORIENTED_EDGE ( 'NONE', *, *, #8684, .T. ) ;
#8315=EDGE_LOOP ( 'NONE', ( #1553, #6676, #11327, #1239 ) ) ;
#8321=DIRECTION ( 'NONE',  ( 0.000000000000000000, 1.000000000000000000, 0.000000000000000000 ) ) ;
#8330=ADVANCED_FACE ( 'NONE', ( #10479 ), #8931, .F. ) ;
#8333=DIRECTION ( 'NONE',  ( -1.000000000000000000, -0.000000000000000000, -0.000000000000000000 ) ) ;
#8336=FACE_BOUND ( 'NONE', #5613, .T. ) ;
#8340=AXIS2_PLACEMENT_3D ( 'NONE', #7000, #2435, #8788 ) ;
#8342=ORIENTED_EDGE ( 'NONE', *, *, #10730, .T. ) ;
#8346=FACE_OUTER_BOUND ( 'NONE', #9050, .T. ) ;
#8353=CIRCLE ( 'NONE', #8171, 1.500000000000001332 ) ;
#8362=ORIENTED_EDGE ( 'NONE', *, *, #8476, .F. ) ;
#8368=EDGE_CURVE ( 'NONE', #2186, #11526, #6191, .T. ) ;
#8371=ORIENTED_EDGE ( 'NONE', *, *, #9746, .T. ) ;
#8379=ORIENTED_EDGE ( 'NONE', *, *, #9813, .F. ) ;
#8386=DIRECTION ( 'NONE',  ( 0.000000000000000000, 1.000000000000000000, 0.000000000000000000 ) ) ;
#8402=EDGE_CURVE ( 'NONE', #9331, #5852, #8650, .T. ) ;
#8414=AXIS2_PLACEMENT_3D ( 'NONE', #11047, #3816, #7484 ) ;
#8428=DIRECTION ( 'NONE',  ( 0.000000000000000000, 0.000000000000000000, 1.000000000000000000 ) ) ;
#8440=AXIS2_PLACEMENT_3D ( 'NONE', #8980, #7790, #3230 ) ;
#8442=CARTESIAN_POINT ( 'NONE',  ( -78.00000000000001421, 59.24264068711927678, 4.242644059037073312 ) ) ;
#8448=CARTESIAN_POINT ( 'NONE',  ( -80.00000000000001421, 46.51471862576140381, -8.485278002320759683 ) ) ;
#8456=EDGE_LOOP ( 'NONE', ( #2784, #7201 ) ) ;
#8465=DIRECTION ( 'NONE',  ( 0.000000000000000000, 1.000000000000000000, 0.000000000000000000 ) ) ;
#8466=CARTESIAN_POINT ( 'NONE',  ( -78.00000000000001421, 67.72792206135787296, 4.242644059037073312 ) ) ;
#8476=EDGE_CURVE ( 'NONE', #1618, #10685, #8838, .T. ) ;
#8482=DIRECTION ( 'NONE',  ( -1.000000000000000000, -0.000000000000000000, -0.000000000000000000 ) ) ;
#8483=ORIENTED_EDGE ( 'NONE', *, *, #3463, .F. ) ;
#8492=DIRECTION ( 'NONE',  ( 0.000000000000000000, 1.000000000000000000, 0.000000000000000000 ) ) ;
#8495=VERTEX_POINT ( 'NONE', #1443 ) ;
#8503=DIRECTION ( 'NONE',  ( 0.000000000000000000, 1.000000000000000000, 0.000000000000000000 ) ) ;
#8504=EDGE_CURVE ( 'NONE', #6038, #10429, #4137, .T. ) ;
#8509=VERTEX_POINT ( 'NONE', #6014 ) ;
#8523=ORIENTED_EDGE ( 'NONE', *, *, #10549, .T. ) ;
#8536=DIRECTION ( 'NONE',  ( -1.000000000000000000, -0.000000000000000000, -0.000000000000000000 ) ) ;
#8539=EDGE_LOOP ( 'NONE', ( #4286, #11538 ) ) ;
#8550=AXIS2_PLACEMENT_3D ( 'NONE', #7796, #4986, #2275 ) ;
#8551=CARTESIAN_POINT ( 'NONE',  ( -78.00000000000002842, 42.27207793864211283, -4.242637315201479353 ) ) ;
#8553=EDGE_LOOP ( 'NONE', ( #8129, #11575 ) ) ;
#8557=AXIS2_PLACEMENT_3D ( 'NONE', #7580, #11206, #10664 ) ;
#8565=CARTESIAN_POINT ( 'NONE',  ( -78.00000000000001421, 67.72792206135787296, -12.72791868944004534 ) ) ;
#8570=VECTOR ( 'NONE', #8045, 1000.000000000000000 ) ;
#8576=EDGE_CURVE ( 'NONE', #7948, #241, #3570, .T. ) ;
#8579=CARTESIAN_POINT ( 'NONE',  ( -80.00000000000001421, 67.72792206135787296, 4.242644059037073312 ) ) ;
#8580=ADVANCED_FACE ( 'NONE', ( #6522 ), #10032, .F. ) ;
#8582=ORIENTED_EDGE ( 'NONE', *, *, #10300, .T. ) ;
#8587=MANIFOLD_SOLID_BREP ( 'Fill Pattern1', #11497 ) ;
#8592=ADVANCED_FACE ( 'NONE', ( #4593 ), #6584, .F. ) ;
#8602=DIRECTION ( 'NONE',  ( 0.000000000000000000, 1.000000000000000000, 0.000000000000000000 ) ) ;
#8616=LINE ( 'NONE', #1359, #4582 ) ;
#8617=ORIENTED_EDGE ( 'NONE', *, *, #8066, .T. ) ;
#8631=VERTEX_POINT ( 'NONE', #3014 ) ;
#8650=CIRCLE ( 'NONE', #1172, 1.500000000000001332 ) ;
#8659=LINE ( 'NONE', #2299, #11699 ) ;
#8663=EDGE_CURVE ( 'NONE', #2384, #8906, #5476, .T. ) ;
#8664=CARTESIAN_POINT ( 'NONE',  ( -80.00000000000002842, 50.75735931288069480, 5.742644059037076865 ) ) ;
#8667=ORIENTED_EDGE ( 'NONE', *, *, #9815, .T. ) ;
#8684=EDGE_CURVE ( 'NONE', #9755, #11556, #9480, .T. ) ;
#8689=FACE_BOUND ( 'NONE', #8456, .T. ) ;
#8690=FACE_BOUND ( 'NONE', #10556, .T. ) ;
#8697=DIRECTION ( 'NONE',  ( 0.000000000000000000, 1.000000000000000000, 0.000000000000000000 ) ) ;
#8699=DIRECTION ( 'NONE',  ( 0.000000000000000000, 1.000000000000000000, 0.000000000000000000 ) ) ;
#8705=EDGE_CURVE ( 'NONE', #8766, #8631, #1269, .T. ) ;
#8707=ORIENTED_EDGE ( 'NONE', *, *, #8663, .F. ) ;
#8722=DIRECTION ( 'NONE',  ( 0.000000000000000000, 1.000000000000000000, 0.000000000000000000 ) ) ;
#8730=CARTESIAN_POINT ( 'NONE',  ( -78.00000000000001421, 50.75735931288069480, -12.72791868944003824 ) ) ;
#8732=DIRECTION ( 'NONE',  ( -1.000000000000000000, -0.000000000000000000, -0.000000000000000000 ) ) ;
#8737=CIRCLE ( 'NONE', #10254, 1.500000000000001332 ) ;
#8738=CYLINDRICAL_SURFACE ( 'NONE', #490, 1.499999999999999556 ) ;
#8750=AXIS2_PLACEMENT_3D ( 'NONE', #4888, #6151, #7822 ) ;
#8755=AXIS2_PLACEMENT_3D ( 'NONE', #8261, #1118, #36 ) ;
#8757=DIRECTION ( 'NONE',  ( 0.000000000000000000, 1.000000000000000000, 0.000000000000000000 ) ) ;
#8758=COLOUR_RGB ( '',0.8941176470588234615, 0.8941176470588234615, 0.8941176470588234615 ) ;
#8760=ORIENTED_EDGE ( 'NONE', *, *, #2416, .T. ) ;
#8764=FACE_OUTER_BOUND ( 'NONE', #4642, .T. ) ;
#8766=VERTEX_POINT ( 'NONE', #11020 ) ;
#8768=DIRECTION ( 'NONE',  ( 0.000000000000000000, 1.000000000000000000, 0.000000000000000000 ) ) ;
#8769=VERTEX_POINT ( 'NONE', #6498 ) ;
#8773=EDGE_CURVE ( 'NONE', #7395, #8040, #7220, .T. ) ;
#8779=EDGE_CURVE ( 'NONE', #6614, #10565, #8737, .T. ) ;
#8781=ORIENTED_EDGE ( 'NONE', *, *, #4863, .T. ) ;
#8785=CIRCLE ( 'NONE', #4961, 1.500000000000001332 ) ;
#8788=DIRECTION ( 'NONE',  ( 0.000000000000000000, 1.000000000000000000, 0.000000000000000000 ) ) ;
#8790=VERTEX_POINT ( 'NONE', #9240 ) ;
#8797=ORIENTED_EDGE ( 'NONE', *, *, #2342, .F. ) ;
#8812=FACE_OUTER_BOUND ( 'NONE', #3417, .T. ) ;
#8815=VECTOR ( 'NONE', #8961, 1000.000000000000000 ) ;
#8818=CARTESIAN_POINT ( 'NONE',  ( -80.00000000000001421, 50.75735931288069480, -4.242637315201482906 ) ) ;
#8821=AXIS2_PLACEMENT_3D ( 'NONE', #6494, #6432, #8280 ) ;
#8838=CIRCLE ( 'NONE', #687, 1.500000000000001332 ) ;
#8850=DIRECTION ( 'NONE',  ( 0.000000000000000000, 1.000000000000000000, 0.000000000000000000 ) ) ;
#8853=ADVANCED_FACE ( 'NONE', ( #8764 ), #11326, .F. ) ;
#8856=ORIENTED_EDGE ( 'NONE', *, *, #447, .F. ) ;
#8860=CARTESIAN_POINT ( 'NONE',  ( -78.00000000000001421, 63.48528137423857487, -8.485278002320759683 ) ) ;
#8863=ORIENTED_EDGE ( 'NONE', *, *, #9812, .F. ) ;
#8865=CARTESIAN_POINT ( 'NONE',  ( -78.00000000000001421, 67.72792206135787296, -12.72791868944004534 ) ) ;
#8868=ORIENTED_EDGE ( 'NONE', *, *, #6760, .F. ) ;
#8872=LINE ( 'NONE', #5451, #4752 ) ;
#8880=EDGE_CURVE ( 'NONE', #5516, #9669, #10055, .T. ) ;
#8896=EDGE_CURVE ( 'NONE', #11337, #1706, #3946, .T. ) ;
#8902=ORIENTED_EDGE ( 'NONE', *, *, #10323, .T. ) ;
#8906=VERTEX_POINT ( 'NONE', #11381 ) ;
#8907=CARTESIAN_POINT ( 'NONE',  ( -78.00000000000001421, 59.24264068711927678, 5.742644059037073312 ) ) ;
#8912=DIRECTION ( 'NONE',  ( -1.000000000000000000, -0.000000000000000000, -0.000000000000000000 ) ) ;
#8913=CARTESIAN_POINT ( 'NONE',  ( -78.00000000000001421, 50.75735931288069480, -4.242637315201482906 ) ) ;
#8918=DIRECTION ( 'NONE',  ( 1.000000000000000000, 0.000000000000000000, 0.000000000000000000 ) ) ;
#8920=VECTOR ( 'NONE', #7723, 1000.000000000000000 ) ;
#8922=ORIENTED_EDGE ( 'NONE', *, *, #839, .F. ) ;
#8923=CARTESIAN_POINT ( 'NONE',  ( -78.00000000000001421, 63.48528137423857487, 9.985284746156350977 ) ) ;
#8931=CYLINDRICAL_SURFACE ( 'NONE', #2133, 1.499999999999999556 ) ;
#8933=LINE ( 'NONE', #7091, #7282 ) ;
#8937=EDGE_LOOP ( 'NONE', ( #1068, #11209 ) ) ;
#8940=CARTESIAN_POINT ( 'NONE',  ( -80.00000000000001421, 50.75735931288069480, -12.72791868944003824 ) ) ;
#8958=EDGE_CURVE ( 'NONE', #6004, #7332, #4923, .T. ) ;
#8961=DIRECTION ( 'NONE',  ( -1.000000000000000000, -0.000000000000000000, -0.000000000000000000 ) ) ;
#8968=LINE ( 'NONE', #10802, #10049 ) ;
#8977=CARTESIAN_POINT ( 'NONE',  ( -78.00000000000000000, 55.00000000000000000, -21.50000000000000000 ) ) ;
#8978=CARTESIAN_POINT ( 'NONE',  ( -78.00000000000002842, 54.99999999999998579, 16.97056612039490986 ) ) ;
#8980=CARTESIAN_POINT ( 'NONE',  ( -78.00000000000001421, 71.97056274847716395, 3.371917795327861178E-06 ) ) ;
#8982=FACE_OUTER_BOUND ( 'NONE', #7198, .T. ) ;
#8989=ORIENTED_EDGE ( 'NONE', *, *, #1408, .T. ) ;
#8995=CIRCLE ( 'NONE', #10509, 1.500000000000001332 ) ;
#8996=ORIENTED_EDGE ( 'NONE', *, *, #6959, .F. ) ;
#9005=ORIENTED_EDGE ( 'NONE', *, *, #8958, .T. ) ;
#9007=CARTESIAN_POINT ( 'NONE',  ( -80.00000000000000000, 55.00000000000000000, 21.50000000000000000 ) ) ;
#9008=CIRCLE ( 'NONE', #3644, 1.500000000000001332 ) ;
#9022=CIRCLE ( 'NONE', #10346, 1.500000000000001332 ) ;
#9040=FACE_BOUND ( 'NONE', #5871, .T. ) ;
#9044=ORIENTED_EDGE ( 'NONE', *, *, #447, .T. ) ;
#9050=EDGE_LOOP ( 'NONE', ( #8238, #9362, #1616, #7940 ) ) ;
#9052=ORIENTED_EDGE ( 'NONE', *, *, #8779, .T. ) ;
#9056=CARTESIAN_POINT ( 'NONE',  ( -80.00000000000001421, 46.51471862576140381, -8.485278002320759683 ) ) ;
#9059=EDGE_CURVE ( 'NONE', #642, #4918, #8353, .T. ) ;
#9066=SHAPE_DEFINITION_REPRESENTATION ( #11212, #3715 ) ;
#9070=AXIS2_PLACEMENT_3D ( 'NONE', #8913, #9804, #6112 ) ;
#9071=EDGE_CURVE ( 'NONE', #8766, #2363, #7604, .T. ) ;
#9076=EDGE_LOOP ( 'NONE', ( #4993, #2338, #10553, #10604 ) ) ;
#9079=EDGE_LOOP ( 'NONE', ( #9052, #4151 ) ) ;
#9088=CYLINDRICAL_SURFACE ( 'NONE', #5360, 1.500000000000000000 ) ;
#9090=ORIENTED_EDGE ( 'NONE', *, *, #8779, .F. ) ;
#9095=CARTESIAN_POINT ( 'NONE',  ( -80.00000000000001421, 50.75735931288069480, -11.22791868944003824 ) ) ;
#9098=ORIENTED_EDGE ( 'NONE', *, *, #10541, .T. ) ;
#9099=DIRECTION ( 'NONE',  ( -1.000000000000000000, -0.000000000000000000, -0.000000000000000000 ) ) ;
#9104=AXIS2_PLACEMENT_3D ( 'NONE', #6946, #6219, #8850 ) ;
#9105=ORIENTED_EDGE ( 'NONE', *, *, #4089, .F. ) ;
#9110=( GEOMETRIC_REPRESENTATION_CONTEXT ( 3 ) GLOBAL_UNCERTAINTY_ASSIGNED_CONTEXT ( ( #3832 ) ) GLOBAL_UNIT_ASSIGNED_CONTEXT ( ( #11105, #9202, #1826 ) ) REPRESENTATION_CONTEXT ( 'NONE', 'WORKASPACE' ) );
#9123=AXIS2_PLACEMENT_3D ( 'NONE', #2931, #9156, #10227 ) ;
#9127=ADVANCED_FACE ( 'NONE', ( #8044 ), #4621, .F. ) ;
#9132=EDGE_LOOP ( 'NONE', ( #8781, #8617 ) ) ;
#9137=EDGE_LOOP ( 'NONE', ( #11011, #9193 ) ) ;
#9140=AXIS2_PLACEMENT_3D ( 'NONE', #6907, #11489, #4259 ) ;
#9146=DIRECTION ( 'NONE',  ( -1.000000000000000000, -0.000000000000000000, -0.000000000000000000 ) ) ;
#9147=CARTESIAN_POINT ( 'NONE',  ( -80.00000000000002842, 42.27207793864211283, -4.242637315201479353 ) ) ;
#9152=DIRECTION ( 'NONE',  ( -1.000000000000000000, -0.000000000000000000, -0.000000000000000000 ) ) ;
#9154=AXIS2_PLACEMENT_3D ( 'NONE', #21, #8244, #3571 ) ;
#9156=DIRECTION ( 'NONE',  ( -1.000000000000000000, -0.000000000000000000, -0.000000000000000000 ) ) ;
#9157=EDGE_CURVE ( 'NONE', #2610, #11481, #314, .T. ) ;
#9162=ORIENTED_EDGE ( 'NONE', *, *, #6760, .T. ) ;
#9191=AXIS2_PLACEMENT_3D ( 'NONE', #7162, #10787, #9780 ) ;
#9192=DIRECTION ( 'NONE',  ( -1.000000000000000000, -0.000000000000000000, -0.000000000000000000 ) ) ;
#9193=ORIENTED_EDGE ( 'NONE', *, *, #2286, .T. ) ;
#9202=( NAMED_UNIT ( * ) PLANE_ANGLE_UNIT ( ) SI_UNIT ( $, .RADIAN. ) );
#9230=DIRECTION ( 'NONE',  ( 0.000000000000000000, 0.000000000000000000, 1.000000000000000000 ) ) ;
#9231=VERTEX_POINT ( 'NONE', #5770 ) ;
#9236=CARTESIAN_POINT ( 'NONE',  ( -78.00000000000002842, 46.51471862576140381, 6.985284746156355418 ) ) ;
#9240=CARTESIAN_POINT ( 'NONE',  ( -80.00000000000002842, 54.99999999999998579, 18.47056612039490986 ) ) ;
#9244=CARTESIAN_POINT ( 'NONE',  ( -80.00000000000002842, 54.99999999999998579, 6.985284746156355418 ) ) ;
#9245=ORIENTED_EDGE ( 'NONE', *, *, #8773, .F. ) ;
#9252=CIRCLE ( 'NONE', #3140, 1.500000000000001332 ) ;
#9256=VERTEX_POINT ( 'NONE', #10365 ) ;
#9259=CARTESIAN_POINT ( 'NONE',  ( -78.00000000000001421, 67.72792206135787296, -4.242637315201482906 ) ) ;
#9265=CARTESIAN_POINT ( 'NONE',  ( -78.00000000000001421, 63.48528137423857487, 3.371917795327861178E-06 ) ) ;
#9266=DIRECTION ( 'NONE',  ( -1.000000000000000000, -0.000000000000000000, -0.000000000000000000 ) ) ;
#9271=DIRECTION ( 'NONE',  ( 0.000000000000000000, 1.000000000000000000, 0.000000000000000000 ) ) ;
#9276=ORIENTED_EDGE ( 'NONE', *, *, #11718, .T. ) ;
#9280=ADVANCED_FACE ( 'NONE', ( #8812 ), #9469, .F. ) ;
#9281=DIRECTION ( 'NONE',  ( -1.000000000000000000, -0.000000000000000000, -0.000000000000000000 ) ) ;
#9284=ORIENTED_EDGE ( 'NONE', *, *, #5592, .T. ) ;
#9288=DIRECTION ( 'NONE',  ( -1.000000000000000000, -0.000000000000000000, -0.000000000000000000 ) ) ;
#9291=EDGE_CURVE ( 'NONE', #43, #1798, #10590, .T. ) ;
#9295=EDGE_CURVE ( 'NONE', #5363, #1831, #3375, .T. ) ;
#9299=DIRECTION ( 'NONE',  ( -1.000000000000000000, -0.000000000000000000, -0.000000000000000000 ) ) ;
#9316=ORIENTED_EDGE ( 'NONE', *, *, #3645, .T. ) ;
#9318=VECTOR ( 'NONE', #7605, 1000.000000000000000 ) ;
#9323=CARTESIAN_POINT ( 'NONE',  ( -78.00000000000001421, 54.99999999999998579, -8.485278002320759683 ) ) ;
#9331=VERTEX_POINT ( 'NONE', #9589 ) ;
#9336=CARTESIAN_POINT ( 'NONE',  ( -80.00000000000001421, 63.48528137423857487, 3.371917795327861178E-06 ) ) ;
#9346=EDGE_CURVE ( 'NONE', #4386, #6519, #4924, .T. ) ;
#9348=DIRECTION ( 'NONE',  ( 0.000000000000000000, 0.000000000000000000, 1.000000000000000000 ) ) ;
#9349=VERTEX_POINT ( 'NONE', #356 ) ;
#9359=ORIENTED_EDGE ( 'NONE', *, *, #1871, .F. ) ;
#9362=ORIENTED_EDGE ( 'NONE', *, *, #10767, .F. ) ;
#9368=CARTESIAN_POINT ( 'NONE',  ( -78.00000000000002842, 46.51471862576140381, 3.371917798797308130E-06 ) ) ;
#9369=ORIENTED_EDGE ( 'NONE', *, *, #1181, .T. ) ;
#9370=FACE_OUTER_BOUND ( 'NONE', #9076, .T. ) ;
#9380=DIRECTION ( 'NONE',  ( -1.000000000000000000, -0.000000000000000000, -0.000000000000000000 ) ) ;
#9383=EDGE_LOOP ( 'NONE', ( #3618, #6972 ) ) ;
#9386=CARTESIAN_POINT ( 'NONE',  ( -80.00000000000001421, 67.72792206135787296, 12.72792543327562775 ) ) ;
#9397=DIRECTION ( 'NONE',  ( 0.000000000000000000, 1.000000000000000000, 0.000000000000000000 ) ) ;
#9400=ORIENTED_EDGE ( 'NONE', *, *, #1731, .F. ) ;
#9402=CIRCLE ( 'NONE', #7691, 21.50000000000000000 ) ;
#9411=ORIENTED_EDGE ( 'NONE', *, *, #9071, .F. ) ;
#9423=DIRECTION ( 'NONE',  ( 0.000000000000000000, 1.000000000000000000, 0.000000000000000000 ) ) ;
#9436=VERTEX_POINT ( 'NONE', #762 ) ;
#9440=DIRECTION ( 'NONE',  ( -1.000000000000000000, -0.000000000000000000, -0.000000000000000000 ) ) ;
#9450=ADVANCED_FACE ( 'NONE', ( #6300 ), #877, .F. ) ;
#9464=ORIENTED_EDGE ( 'NONE', *, *, #5592, .F. ) ;
#9469=CYLINDRICAL_SURFACE ( 'NONE', #1839, 1.500000000000000000 ) ;
#9476=EDGE_LOOP ( 'NONE', ( #1740, #9090, #3202, #9276 ) ) ;
#9480=LINE ( 'NONE', #6622, #6439 ) ;
#9487=AXIS2_PLACEMENT_3D ( 'NONE', #9551, #5849, #5010 ) ;
#9491=AXIS2_PLACEMENT_3D ( 'NONE', #4839, #10983, #2853 ) ;
#9492=VERTEX_POINT ( 'NONE', #11668 ) ;
#9494=LINE ( 'NONE', #9557, #9931 ) ;
#9497=ORIENTED_EDGE ( 'NONE', *, *, #5169, .F. ) ;
#9500=FACE_OUTER_BOUND ( 'NONE', #10701, .T. ) ;
#9503=LINE ( 'NONE', #2072, #11076 ) ;
#9507=EDGE_CURVE ( 'NONE', #3587, #10459, #11793, .T. ) ;
#9510=DIRECTION ( 'NONE',  ( -1.000000000000000000, -0.000000000000000000, -0.000000000000000000 ) ) ;
#9515=FACE_OUTER_BOUND ( 'NONE', #7209, .T. ) ;
#9522=CIRCLE ( 'NONE', #11612, 1.500000000000001332 ) ;
#9524=FACE_BOUND ( 'NONE', #1046, .T. ) ;
#9531=CARTESIAN_POINT ( 'NONE',  ( -78.00000000000002842, 42.27207793864211283, -5.742637315201479353 ) ) ;
#9551=CARTESIAN_POINT ( 'NONE',  ( -78.00000000000002842, 50.75735931288069480, 4.242644059037076865 ) ) ;
#9556=FACE_OUTER_BOUND ( 'NONE', #1539, .T. ) ;
#9557=CARTESIAN_POINT ( 'NONE',  ( -78.00000000000001421, 67.72792206135787296, -11.22791868944004534 ) ) ;
#9584=FACE_BOUND ( 'NONE', #9137, .T. ) ;
#9585=ORIENTED_EDGE ( 'NONE', *, *, #1460, .T. ) ;
#9588=FACE_OUTER_BOUND ( 'NONE', #11183, .T. ) ;
#9589=CARTESIAN_POINT ( 'NONE',  ( -78.00000000000001421, 67.72792206135787296, 2.742644059037073312 ) ) ;
#9593=CIRCLE ( 'NONE', #8068, 1.500000000000001332 ) ;
#9597=CYLINDRICAL_SURFACE ( 'NONE', #6159, 1.500000000000000000 ) ;
#9599=EDGE_CURVE ( 'NONE', #5447, #3221, #9879, .T. ) ;
#9604=DIRECTION ( 'NONE',  ( -1.000000000000000000, -0.000000000000000000, -0.000000000000000000 ) ) ;
#9614=EDGE_CURVE ( 'NONE', #911, #4578, #3384, .T. ) ;
#9615=ORIENTED_EDGE ( 'NONE', *, *, #11568, .T. ) ;
#9621=CARTESIAN_POINT ( 'NONE',  ( -78.00000000000002842, 59.24264068711927678, 12.72792543327563131 ) ) ;
#9624=ORIENTED_EDGE ( 'NONE', *, *, #6177, .F. ) ;
#9626=CARTESIAN_POINT ( 'NONE',  ( -80.00000000000001421, 59.24264068711927678, -4.242637315201482906 ) ) ;
#9627=DIRECTION ( 'NONE',  ( -1.000000000000000000, -0.000000000000000000, -0.000000000000000000 ) ) ;
#9639=FACE_BOUND ( 'NONE', #4264, .T. ) ;
#9645=EDGE_CURVE ( 'NONE', #2363, #11604, #3703, .T. ) ;
#9646=CARTESIAN_POINT ( 'NONE',  ( -80.00000000000001421, 59.24264068711927678, 5.742644059037073312 ) ) ;
#9647=ORIENTED_EDGE ( 'NONE', *, *, #9291, .T. ) ;
#9651=CARTESIAN_POINT ( 'NONE',  ( -80.00000000000001421, 46.51471862576140381, -9.985278002320759683 ) ) ;
#9660=EDGE_LOOP ( 'NONE', ( #1767, #3485, #4823, #6500 ) ) ;
#9669=VERTEX_POINT ( 'NONE', #11116 ) ;
#9678=CIRCLE ( 'NONE', #8340, 1.500000000000001332 ) ;
#9679=EDGE_CURVE ( 'NONE', #6194, #9256, #1423, .T. ) ;
#9685=CARTESIAN_POINT ( 'NONE',  ( -78.00000000000001421, 59.24264068711927678, -5.742637315201482906 ) ) ;
#9687=ORIENTED_EDGE ( 'NONE', *, *, #11176, .F. ) ;
#9691=DIRECTION ( 'NONE',  ( 0.000000000000000000, 1.000000000000000000, 0.000000000000000000 ) ) ;
#9698=FACE_BOUND ( 'NONE', #1393, .T. ) ;
#9701=CARTESIAN_POINT ( 'NONE',  ( -78.00000000000002842, 50.75735931288069480, 4.242644059037076865 ) ) ;
#9704=CARTESIAN_POINT ( 'NONE',  ( -78.00000000000002842, 42.27207793864211283, -4.242637315201479353 ) ) ;
#9720=CARTESIAN_POINT ( 'NONE',  ( -78.00000000000002842, 54.99999999999998579, 8.485284746156354529 ) ) ;
#9724=ORIENTED_EDGE ( 'NONE', *, *, #1765, .T. ) ;
#9725=DIRECTION ( 'NONE',  ( -1.000000000000000000, -0.000000000000000000, -0.000000000000000000 ) ) ;
#9731=VECTOR ( 'NONE', #581, 1000.000000000000000 ) ;
#9732=AXIS2_PLACEMENT_3D ( 'NONE', #2738, #805, #1818 ) ;
#9737=FACE_OUTER_BOUND ( 'NONE', #5430, .T. ) ;
#9745=FACE_OUTER_BOUND ( 'NONE', #7300, .T. ) ;
#9746=EDGE_CURVE ( 'NONE', #11526, #19, #1088, .T. ) ;
#9751=CARTESIAN_POINT ( 'NONE',  ( -78.00000000000001421, 63.48528137423857487, -8.485278002320759683 ) ) ;
#9752=CARTESIAN_POINT ( 'NONE',  ( -78.00000000000002842, 54.99999999999998579, 6.985284746156355418 ) ) ;
#9753=AXIS2_PLACEMENT_3D ( 'NONE', #9826, #2527, #1615 ) ;
#9755=VERTEX_POINT ( 'NONE', #9685 ) ;
#9770=AXIS2_PLACEMENT_3D ( 'NONE', #3049, #2932, #6600 ) ;
#9773=DIRECTION ( 'NONE',  ( 0.000000000000000000, 0.000000000000000000, 1.000000000000000000 ) ) ;
#9780=DIRECTION ( 'NONE',  ( 0.000000000000000000, 1.000000000000000000, 0.000000000000000000 ) ) ;
#9787=VERTEX_POINT ( 'NONE', #4178 ) ;
#9788=CARTESIAN_POINT ( 'NONE',  ( -78.00000000000001421, 50.75735931288069480, -4.242637315201482906 ) ) ;
#9790=EDGE_LOOP ( 'NONE', ( #484, #8362, #6245, #5137 ) ) ;
#9797=EDGE_CURVE ( 'NONE', #8631, #11604, #8179, .T. ) ;
#9803=DIRECTION ( 'NONE',  ( 0.000000000000000000, 1.000000000000000000, 0.000000000000000000 ) ) ;
#9804=DIRECTION ( 'NONE',  ( -1.000000000000000000, -0.000000000000000000, -0.000000000000000000 ) ) ;
#9808=FACE_OUTER_BOUND ( 'NONE', #1651, .T. ) ;
#9811=FACE_BOUND ( 'NONE', #7629, .T. ) ;
#9812=EDGE_CURVE ( 'NONE', #4918, #4978, #5086, .T. ) ;
#9813=EDGE_CURVE ( 'NONE', #1264, #8509, #11603, .T. ) ;
#9815=EDGE_CURVE ( 'NONE', #10744, #8509, #6887, .T. ) ;
#9819=CYLINDRICAL_SURFACE ( 'NONE', #2649, 1.500000000000000000 ) ;
#9822=EDGE_CURVE ( 'NONE', #4492, #8007, #3586, .T. ) ;
#9826=CARTESIAN_POINT ( 'NONE',  ( -78.00000000000001421, 46.51471862576140381, -8.485278002320759683 ) ) ;
#9829=DIRECTION ( 'NONE',  ( 0.000000000000000000, 1.000000000000000000, 0.000000000000000000 ) ) ;
#9835=FACE_OUTER_BOUND ( 'NONE', #7019, .T. ) ;
#9837=ORIENTED_EDGE ( 'NONE', *, *, #10967, .F. ) ;
#9842=CARTESIAN_POINT ( 'NONE',  ( -78.00000000000002842, 59.24264068711927678, 12.72792543327563131 ) ) ;
#9850=AXIS2_PLACEMENT_3D ( 'NONE', #5806, #452, #8492 ) ;
#9851=ORIENTED_EDGE ( 'NONE', *, *, #3740, .F. ) ;
#9866=DIRECTION ( 'NONE',  ( -1.000000000000000000, -0.000000000000000000, -0.000000000000000000 ) ) ;
#9873=VERTEX_POINT ( 'NONE', #11354 ) ;
#9874=CARTESIAN_POINT ( 'NONE',  ( -78.00000000000001421, 59.24264068711927678, -4.242637315201482906 ) ) ;
#9879=CIRCLE ( 'NONE', #5884, 1.500000000000001332 ) ;
#9888=DIRECTION ( 'NONE',  ( 0.000000000000000000, 1.000000000000000000, 0.000000000000000000 ) ) ;
#9890=CARTESIAN_POINT ( 'NONE',  ( -78.00000000000002842, 42.27207793864211283, 4.242644059037075976 ) ) ;
#9891=VECTOR ( 'NONE', #5017, 1000.000000000000000 ) ;
#9897=LINE ( 'NONE', #6205, #2112 ) ;
#9901=AXIS2_PLACEMENT_3D ( 'NONE', #1202, #10118, #9230 ) ;
#9906=VERTEX_POINT ( 'NONE', #11528 ) ;
#9910=ORIENTED_EDGE ( 'NONE', *, *, #3072, .F. ) ;
#9914=CARTESIAN_POINT ( 'NONE',  ( -80.00000000000001421, 67.72792206135787296, -14.22791868944004356 ) ) ;
#9923=DIRECTION ( 'NONE',  ( -1.000000000000000000, -0.000000000000000000, -0.000000000000000000 ) ) ;
#9931=VECTOR ( 'NONE', #1285, 1000.000000000000000 ) ;
#9943=EDGE_LOOP ( 'NONE', ( #9851, #8760, #2792, #5049 ) ) ;
#9950=ORIENTED_EDGE ( 'NONE', *, *, #2693, .F. ) ;
#9959=AXIS2_PLACEMENT_3D ( 'NONE', #3311, #6079, #5287 ) ;
#9972=EDGE_LOOP ( 'NONE', ( #11731, #6950, #1699, #4082 ) ) ;
#9975=ORIENTED_EDGE ( 'NONE', *, *, #8008, .F. ) ;
#10013=CIRCLE ( 'NONE', #4872, 1.500000000000001332 ) ;
#10032=CYLINDRICAL_SURFACE ( 'NONE', #4911, 1.500000000000000000 ) ;
#10034=DIRECTION ( 'NONE',  ( -1.000000000000000000, -0.000000000000000000, -0.000000000000000000 ) ) ;
#10035=FACE_OUTER_BOUND ( 'NONE', #1214, .T. ) ;
#10046=CARTESIAN_POINT ( 'NONE',  ( -78.00000000000001421, 46.51471862576140381, -9.985278002320759683 ) ) ;
#10047=CARTESIAN_POINT ( 'NONE',  ( -80.00000000000002842, 46.51471862576140381, 8.485284746156354529 ) ) ;
#10049=VECTOR ( 'NONE', #7176, 1000.000000000000000 ) ;
#10055=CIRCLE ( 'NONE', #6075, 1.500000000000001332 ) ;
#10058=AXIS2_PLACEMENT_3D ( 'NONE', #9368, #5070, #258 ) ;
#10060=EDGE_LOOP ( 'NONE', ( #571, #6446 ) ) ;
#10064=FACE_OUTER_BOUND ( 'NONE', #10120, .T. ) ;
#10067=VECTOR ( 'NONE', #9266, 1000.000000000000000 ) ;
#10069=AXIS2_PLACEMENT_3D ( 'NONE', #2992, #2023, #9397 ) ;
#10072=EDGE_LOOP ( 'NONE', ( #4989, #704, #4235, #8523 ) ) ;
#10086=ORIENTED_EDGE ( 'NONE', *, *, #11568, .F. ) ;
#10091=LINE ( 'NONE', #28, #4403 ) ;
#10094=ORIENTED_EDGE ( 'NONE', *, *, #1408, .F. ) ;
#10110=CIRCLE ( 'NONE', #3044, 1.500000000000001332 ) ;
#10111=ORIENTED_EDGE ( 'NONE', *, *, #4925, .F. ) ;
#10113=AXIS2_PLACEMENT_3D ( 'NONE', #6766, #6705, #3932 ) ;
#10118=DIRECTION ( 'NONE',  ( -1.000000000000000000, -0.000000000000000000, -0.000000000000000000 ) ) ;
#10120=EDGE_LOOP ( 'NONE', ( #8856, #6095, #4414, #11463 ) ) ;
#10123=DIRECTION ( 'NONE',  ( 0.000000000000000000, 0.000000000000000000, 1.000000000000000000 ) ) ;
#10126=CIRCLE ( 'NONE', #4025, 1.500000000000001332 ) ;
#10132=ORIENTED_EDGE ( 'NONE', *, *, #10975, .T. ) ;
#10134=AXIS2_PLACEMENT_3D ( 'NONE', #8001, #7114, #7056 ) ;
#10139=VECTOR ( 'NONE', #29, 1000.000000000000000 ) ;
#10142=ORIENTED_EDGE ( 'NONE', *, *, #4890, .F. ) ;
#10154=CARTESIAN_POINT ( 'NONE',  ( -78.00000000000002842, 54.99999999999998579, 9.985284746156354529 ) ) ;
#10155=CARTESIAN_POINT ( 'NONE',  ( -78.00000000000001421, 63.48528137423857487, -1.499996628082204797 ) ) ;
#10156=ADVANCED_FACE ( 'NONE', ( #3017 ), #1091, .F. ) ;
#10163=CARTESIAN_POINT ( 'NONE',  ( -80.00000000000001421, 59.24264068711927678, -2.742637315201482462 ) ) ;
#10167=EDGE_LOOP ( 'NONE', ( #9950, #3214 ) ) ;
#10169=CARTESIAN_POINT ( 'NONE',  ( -78.00000000000001421, 50.75735931288069480, -11.22791868944003824 ) ) ;
#10170=LINE ( 'NONE', #11786, #195 ) ;
#10171=CARTESIAN_POINT ( 'NONE',  ( -80.00000000000001421, 54.99999999999998579, -9.985278002320759683 ) ) ;
#10175=EDGE_LOOP ( 'NONE', ( #152, #11059 ) ) ;
#10176=ADVANCED_FACE ( 'NONE', ( #6802 ), #1149, .F. ) ;
#10177=EDGE_CURVE ( 'NONE', #7683, #322, #2439, .T. ) ;
#10187=EDGE_LOOP ( 'NONE', ( #9400, #10199, #8232, #5554 ) ) ;
#10188=EDGE_CURVE ( 'NONE', #1033, #6241, #1857, .T. ) ;
#10199=ORIENTED_EDGE ( 'NONE', *, *, #11357, .T. ) ;
#10203=CYLINDRICAL_SURFACE ( 'NONE', #1381, 1.500000000000000000 ) ;
#10216=CARTESIAN_POINT ( 'NONE',  ( -78.00000000000002842, 42.27207793864211283, -2.742637315201478909 ) ) ;
#10217=FACE_OUTER_BOUND ( 'NONE', #715, .T. ) ;
#10218=ORIENTED_EDGE ( 'NONE', *, *, #8135, .T. ) ;
#10226=EDGE_LOOP ( 'NONE', ( #6202, #1070, #404, #7524 ) ) ;
#10227=DIRECTION ( 'NONE',  ( 0.000000000000000000, 1.000000000000000000, 0.000000000000000000 ) ) ;
#10238=CARTESIAN_POINT ( 'NONE',  ( -78.00000000000001421, 67.72792206135787296, 2.742644059037073312 ) ) ;
#10246=FACE_BOUND ( 'NONE', #6804, .T. ) ;
#10247=ADVANCED_FACE ( 'NONE', ( #9835 ), #3606, .T. ) ;
#10251=CARTESIAN_POINT ( 'NONE',  ( -78.00000000000001421, 42.27207793864211283, -11.22791868944003824 ) ) ;
#10252=ORIENTED_EDGE ( 'NONE', *, *, #8663, .T. ) ;
#10253=DIRECTION ( 'NONE',  ( 0.000000000000000000, 0.000000000000000000, 1.000000000000000000 ) ) ;
#10254=AXIS2_PLACEMENT_3D ( 'NONE', #2169, #1930, #8285 ) ;
#10257=ORIENTED_EDGE ( 'NONE', *, *, #206, .T. ) ;
#10279=EDGE_CURVE ( 'NONE', #9873, #10795, #11743, .T. ) ;
#10290=CARTESIAN_POINT ( 'NONE',  ( -78.00000000000002842, 50.75735931288069480, 12.72792543327563131 ) ) ;
#10291=FACE_OUTER_BOUND ( 'NONE', #5779, .T. ) ;
#10292=CARTESIAN_POINT ( 'NONE',  ( -80.00000000000001421, 63.48528137423857487, 9.985284746156350977 ) ) ;
#10300=EDGE_CURVE ( 'NONE', #5239, #10429, #9522, .T. ) ;
#10303=CARTESIAN_POINT ( 'NONE',  ( -78.00000000000001421, 59.24264068711927678, 2.742644059037073312 ) ) ;
#10307=VECTOR ( 'NONE', #11649, 1000.000000000000000 ) ;
#10308=FACE_OUTER_BOUND ( 'NONE', #4570, .T. ) ;
#10313=CARTESIAN_POINT ( 'NONE',  ( -80.00000000000002842, 54.99999999999998579, 8.485284746156354529 ) ) ;
#10314=CIRCLE ( 'NONE', #172, 1.500000000000001332 ) ;
#10317=CARTESIAN_POINT ( 'NONE',  ( -78.00000000000001421, 67.72792206135787296, -5.742637315201482906 ) ) ;
#10318=VERTEX_POINT ( 'NONE', #8107 ) ;
#10323=EDGE_CURVE ( 'NONE', #1033, #1850, #7217, .T. ) ;
#10346=AXIS2_PLACEMENT_3D ( 'NONE', #2229, #4875, #11263 ) ;
#10349=ORIENTED_EDGE ( 'NONE', *, *, #3751, .T. ) ;
#10352=CYLINDRICAL_SURFACE ( 'NONE', #7552, 1.499999999999999556 ) ;
#10358=CIRCLE ( 'NONE', #4816, 1.500000000000001332 ) ;
#10360=FACE_BOUND ( 'NONE', #731, .T. ) ;
#10365=CARTESIAN_POINT ( 'NONE',  ( -80.00000000000000000, 54.99999999999999289, 1.500003371917797201 ) ) ;
#10367=ORIENTED_EDGE ( 'NONE', *, *, #6293, .F. ) ;
#10371=ORIENTED_EDGE ( 'NONE', *, *, #2334, .F. ) ;
#10376=ORIENTED_EDGE ( 'NONE', *, *, #3103, .F. ) ;
#10386=ORIENTED_EDGE ( 'NONE', *, *, #2334, .T. ) ;
#10394=DIRECTION ( 'NONE',  ( -1.000000000000000000, -0.000000000000000000, -0.000000000000000000 ) ) ;
#10400=ADVANCED_FACE ( 'NONE', ( #893 ), #5588, .F. ) ;
#10404=ORIENTED_EDGE ( 'NONE', *, *, #11012, .F. ) ;
#10413=ORIENTED_EDGE ( 'NONE', *, *, #5587, .T. ) ;
#10418=CARTESIAN_POINT ( 'NONE',  ( -78.00000000000002842, 46.51471862576140381, 3.371917798797308130E-06 ) ) ;
#10419=DIRECTION ( 'NONE',  ( -1.000000000000000000, -0.000000000000000000, -0.000000000000000000 ) ) ;
#10429=VERTEX_POINT ( 'NONE', #11192 ) ;
#10443=ORIENTED_EDGE ( 'NONE', *, *, #2922, .T. ) ;
#10451=ORIENTED_EDGE ( 'NONE', *, *, #5820, .F. ) ;
#10453=LINE ( 'NONE', #6713, #8920 ) ;
#10454=DIRECTION ( 'NONE',  ( -1.000000000000000000, -0.000000000000000000, -0.000000000000000000 ) ) ;
#10456=DIRECTION ( 'NONE',  ( 0.000000000000000000, 1.000000000000000000, 0.000000000000000000 ) ) ;
#10459=VERTEX_POINT ( 'NONE', #10303 ) ;
#10461=DIRECTION ( 'NONE',  ( 0.000000000000000000, 0.000000000000000000, 1.000000000000000000 ) ) ;
#10462=ADVANCED_FACE ( 'NONE', ( #1919 ), #5646, .F. ) ;
#10463=CARTESIAN_POINT ( 'NONE',  ( -78.00000000000001421, 71.97056274847716395, -1.499996628082204797 ) ) ;
#10469=FACE_OUTER_BOUND ( 'NONE', #6567, .T. ) ;
#10470=CARTESIAN_POINT ( 'NONE',  ( -78.00000000000001421, 59.24264068711928388, -11.22791868944003824 ) ) ;
#10471=AXIS2_PLACEMENT_3D ( 'NONE', #4018, #5642, #1251 ) ;
#10476=CARTESIAN_POINT ( 'NONE',  ( -78.00000000000001421, 67.72792206135787296, -5.742637315201482906 ) ) ;
#10479=FACE_OUTER_BOUND ( 'NONE', #2353, .T. ) ;
#10501=DIRECTION ( 'NONE',  ( -1.000000000000000000, -0.000000000000000000, -0.000000000000000000 ) ) ;
#10509=AXIS2_PLACEMENT_3D ( 'NONE', #5326, #8252, #4541 ) ;
#10510=DIRECTION ( 'NONE',  ( 0.000000000000000000, 1.000000000000000000, 0.000000000000000000 ) ) ;
#10515=CARTESIAN_POINT ( 'NONE',  ( -78.00000000000002842, 46.51471862576140381, 9.985284746156354529 ) ) ;
#10517=ORIENTED_EDGE ( 'NONE', *, *, #5055, .T. ) ;
#10534=CARTESIAN_POINT ( 'NONE',  ( -78.00000000000001421, 67.72792206135787296, 11.22792543327562775 ) ) ;
#10541=EDGE_CURVE ( 'NONE', #8040, #3221, #11134, .T. ) ;
#10549=EDGE_CURVE ( 'NONE', #7713, #6771, #3023, .T. ) ;
#10553=ORIENTED_EDGE ( 'NONE', *, *, #6263, .T. ) ;
#10556=EDGE_LOOP ( 'NONE', ( #10808, #9687 ) ) ;
#10558=DIRECTION ( 'NONE',  ( -1.000000000000000000, -0.000000000000000000, -0.000000000000000000 ) ) ;
#10559=DIRECTION ( 'NONE',  ( 0.000000000000000000, 1.000000000000000000, 0.000000000000000000 ) ) ;
#10565=VERTEX_POINT ( 'NONE', #2277 ) ;
#10568=DIRECTION ( 'NONE',  ( -1.000000000000000000, -0.000000000000000000, -0.000000000000000000 ) ) ;
#10570=ORIENTED_EDGE ( 'NONE', *, *, #1332, .F. ) ;
#10572=CARTESIAN_POINT ( 'NONE',  ( -80.00000000000002842, 42.27207793864211283, 5.742644059037075088 ) ) ;
#10573=DIRECTION ( 'NONE',  ( -1.000000000000000000, -0.000000000000000000, -0.000000000000000000 ) ) ;
#10574=CARTESIAN_POINT ( 'NONE',  ( -78.00000000000001421, 67.72792206135787296, -14.22791868944004356 ) ) ;
#10590=LINE ( 'NONE', #2391, #6270 ) ;
#10595=DIRECTION ( 'NONE',  ( -1.000000000000000000, -0.000000000000000000, -0.000000000000000000 ) ) ;
#10599=VERTEX_POINT ( 'NONE', #9646 ) ;
#10603=CARTESIAN_POINT ( 'NONE',  ( -78.00000000000001421, 63.48528137423857487, -6.985278002320760571 ) ) ;
#10604=ORIENTED_EDGE ( 'NONE', *, *, #7210, .F. ) ;
#10607=LINE ( 'NONE', #5179, #2694 ) ;
#10611=DIRECTION ( 'NONE',  ( 0.000000000000000000, 1.000000000000000000, 0.000000000000000000 ) ) ;
#10625=DIRECTION ( 'NONE',  ( 0.000000000000000000, 0.000000000000000000, 1.000000000000000000 ) ) ;
#10636=EDGE_LOOP ( 'NONE', ( #626, #3039 ) ) ;
#10644=VECTOR ( 'NONE', #5760, 1000.000000000000000 ) ;
#10649=DIRECTION ( 'NONE',  ( 0.000000000000000000, 0.000000000000000000, 1.000000000000000000 ) ) ;
#10654=VERTEX_POINT ( 'NONE', #10476 ) ;
#10655=EDGE_CURVE ( 'NONE', #10795, #1798, #3789, .T. ) ;
#10656=DIRECTION ( 'NONE',  ( -1.000000000000000000, -0.000000000000000000, -0.000000000000000000 ) ) ;
#10661=DIRECTION ( 'NONE',  ( -1.000000000000000000, -0.000000000000000000, -0.000000000000000000 ) ) ;
#10664=DIRECTION ( 'NONE',  ( 0.000000000000000000, 0.000000000000000000, 1.000000000000000000 ) ) ;
#10666=ORIENTED_EDGE ( 'NONE', *, *, #3274, .T. ) ;
#10677=EDGE_LOOP ( 'NONE', ( #9105, #9615, #5509, #7968 ) ) ;
#10683=ADVANCED_FACE ( 'NONE', ( #7682 ), #6792, .T. ) ;
#10685=VERTEX_POINT ( 'NONE', #9531 ) ;
#10693=AXIS2_PLACEMENT_3D ( 'NONE', #3269, #11226, #4108 ) ;
#10701=EDGE_LOOP ( 'NONE', ( #2437, #9245, #7316, #4214 ) ) ;
#10709=DIRECTION ( 'NONE',  ( 0.000000000000000000, 1.000000000000000000, 0.000000000000000000 ) ) ;
#10714=CYLINDRICAL_SURFACE ( 'NONE', #9753, 1.499999999999999556 ) ;
#10715=EDGE_LOOP ( 'NONE', ( #5889, #5624, #6405, #9624 ) ) ;
#10716=CARTESIAN_POINT ( 'NONE',  ( -78.00000000000001421, 71.97056274847716395, 3.371917795327861178E-06 ) ) ;
#10717=AXIS2_PLACEMENT_3D ( 'NONE', #3785, #9288, #4510 ) ;
#10722=DIRECTION ( 'NONE',  ( -1.000000000000000000, -0.000000000000000000, -0.000000000000000000 ) ) ;
#10726=DIRECTION ( 'NONE',  ( 0.000000000000000000, 1.000000000000000000, 0.000000000000000000 ) ) ;
#10727=ORIENTED_EDGE ( 'NONE', *, *, #8402, .F. ) ;
#10728=CARTESIAN_POINT ( 'NONE',  ( -78.00000000000001421, 67.72792206135787296, 14.22792543327562775 ) ) ;
#10730=EDGE_CURVE ( 'NONE', #2349, #6004, #2393, .T. ) ;
#10734=AXIS2_PLACEMENT_3D ( 'NONE', #2525, #3300, #3353 ) ;
#10737=CARTESIAN_POINT ( 'NONE',  ( -80.00000000000002842, 46.51471862576140381, 1.500003371917798756 ) ) ;
#10744=VERTEX_POINT ( 'NONE', #2458 ) ;
#10756=CARTESIAN_POINT ( 'NONE',  ( -80.00000000000001421, 67.72792206135787296, 11.22792543327562775 ) ) ;
#10764=CARTESIAN_POINT ( 'NONE',  ( -78.00000000000001421, 46.51471862576140381, -8.485278002320759683 ) ) ;
#10767=EDGE_CURVE ( 'NONE', #5641, #9755, #7244, .T. ) ;
#10772=DIRECTION ( 'NONE',  ( 0.000000000000000000, 0.000000000000000000, 1.000000000000000000 ) ) ;
#10787=DIRECTION ( 'NONE',  ( -1.000000000000000000, -0.000000000000000000, -0.000000000000000000 ) ) ;
#10795=VERTEX_POINT ( 'NONE', #5277 ) ;
#10798=VECTOR ( 'NONE', #6203, 1000.000000000000000 ) ;
#10802=CARTESIAN_POINT ( 'NONE',  ( -78.00000000000001421, 63.48528137423857487, 6.985284746156351865 ) ) ;
#10804=DIRECTION ( 'NONE',  ( 0.000000000000000000, 1.000000000000000000, 0.000000000000000000 ) ) ;
#10808=ORIENTED_EDGE ( 'NONE', *, *, #8958, .F. ) ;
#10812=LINE ( 'NONE', #5267, #8027 ) ;
#10818=CYLINDRICAL_SURFACE ( 'NONE', #11451, 1.499999999999999556 ) ;
#10823=CARTESIAN_POINT ( 'NONE',  ( -80.00000000000001421, 54.99999999999999289, -15.47055937655931501 ) ) ;
#10829=CARTESIAN_POINT ( 'NONE',  ( -78.00000000000001421, 63.48528137423857487, 3.371917795327861178E-06 ) ) ;
#10834=VECTOR ( 'NONE', #2341, 1000.000000000000000 ) ;
#10836=ORIENTED_EDGE ( 'NONE', *, *, #1525, .T. ) ;
#10850=DIRECTION ( 'NONE',  ( -1.000000000000000000, -0.000000000000000000, -0.000000000000000000 ) ) ;
#10857=LINE ( 'NONE', #7286, #8815 ) ;
#10865=DIRECTION ( 'NONE',  ( 0.000000000000000000, 0.000000000000000000, -1.000000000000000000 ) ) ;
#10867=VERTEX_POINT ( 'NONE', #880 ) ;
#10871=CIRCLE ( 'NONE', #2274, 1.500000000000001332 ) ;
#10879=EDGE_CURVE ( 'NONE', #10459, #3494, #1670, .T. ) ;
#10880=CIRCLE ( 'NONE', #554, 1.500000000000001332 ) ;
#10883=AXIS2_PLACEMENT_3D ( 'NONE', #5329, #7964, #7191 ) ;
#10893=VECTOR ( 'NONE', #1564, 1000.000000000000000 ) ;
#10901=AXIS2_PLACEMENT_3D ( 'NONE', #7581, #2901, #9423 ) ;
#10908=CYLINDRICAL_SURFACE ( 'NONE', #1183, 1.499999999999999556 ) ;
#10910=ADVANCED_FACE ( 'NONE', ( #7202 ), #9819, .F. ) ;
#10926=ORIENTED_EDGE ( 'NONE', *, *, #7423, .T. ) ;
#10927=LINE ( 'NONE', #8907, #10307 ) ;
#10936=DIRECTION ( 'NONE',  ( -1.000000000000000000, -0.000000000000000000, -0.000000000000000000 ) ) ;
#10945=CYLINDRICAL_SURFACE ( 'NONE', #3074, 1.500000000000000000 ) ;
#10951=ORIENTED_EDGE ( 'NONE', *, *, #8504, .F. ) ;
#10967=EDGE_CURVE ( 'NONE', #9436, #19, #8872, .T. ) ;
#10968=CARTESIAN_POINT ( 'NONE',  ( -78.00000000000001421, 54.99999999999998579, -9.985278002320759683 ) ) ;
#10972=ORIENTED_EDGE ( 'NONE', *, *, #6827, .F. ) ;
#10975=EDGE_CURVE ( 'NONE', #96, #4662, #4552, .T. ) ;
#10983=DIRECTION ( 'NONE',  ( -1.000000000000000000, -0.000000000000000000, -0.000000000000000000 ) ) ;
#10995=EDGE_CURVE ( 'NONE', #5852, #9331, #6297, .T. ) ;
#11002=ORIENTED_EDGE ( 'NONE', *, *, #11272, .F. ) ;
#11004=ORIENTED_EDGE ( 'NONE', *, *, #8880, .F. ) ;
#11011=ORIENTED_EDGE ( 'NONE', *, *, #7065, .T. ) ;
#11012=EDGE_CURVE ( 'NONE', #6194, #1492, #2818, .T. ) ;
#11015=CYLINDRICAL_SURFACE ( 'NONE', #7110, 1.499999999999999556 ) ;
#11019=VECTOR ( 'NONE', #4116, 1000.000000000000000 ) ;
#11020=CARTESIAN_POINT ( 'NONE',  ( -78.00000000000001421, 42.27207793864211283, -11.22791868944003824 ) ) ;
#11021=AXIS2_PLACEMENT_3D ( 'NONE', #1061, #282, #7433 ) ;
#11022=ORIENTED_EDGE ( 'NONE', *, *, #8576, .F. ) ;
#11025=DIRECTION ( 'NONE',  ( -1.000000000000000000, -0.000000000000000000, -0.000000000000000000 ) ) ;
#11026=EDGE_CURVE ( 'NONE', #6771, #7713, #3776, .T. ) ;
#11033=( NAMED_UNIT ( * ) PLANE_ANGLE_UNIT ( ) SI_UNIT ( $, .RADIAN. ) );
#11040=ORIENTED_EDGE ( 'NONE', *, *, #3370, .F. ) ;
#11047=CARTESIAN_POINT ( 'NONE',  ( -78.00000000000002842, 38.02943725152282184, 3.371917797929946392E-06 ) ) ;
#11054=EDGE_CURVE ( 'NONE', #10565, #6614, #4931, .T. ) ;
#11059=ORIENTED_EDGE ( 'NONE', *, *, #2201, .T. ) ;
#11060=DIRECTION ( 'NONE',  ( -1.000000000000000000, -0.000000000000000000, -0.000000000000000000 ) ) ;
#11063=DIRECTION ( 'NONE',  ( -1.000000000000000000, -0.000000000000000000, -0.000000000000000000 ) ) ;
#11076=VECTOR ( 'NONE', #9380, 1000.000000000000000 ) ;
#11086=ORIENTED_EDGE ( 'NONE', *, *, #2937, .F. ) ;
#11088=CYLINDRICAL_SURFACE ( 'NONE', #572, 1.499999999999999556 ) ;
#11091=VECTOR ( 'NONE', #4822, 1000.000000000000000 ) ;
#11093=DIRECTION ( 'NONE',  ( 0.000000000000000000, 1.000000000000000000, 0.000000000000000000 ) ) ;
#11097=ORIENTED_EDGE ( 'NONE', *, *, #2480, .F. ) ;
#11105=( LENGTH_UNIT ( ) NAMED_UNIT ( * ) SI_UNIT ( .MILLI., .METRE. ) );
#11116=CARTESIAN_POINT ( 'NONE',  ( -80.00000000000001421, 50.75735931288069480, -2.742637315201482462 ) ) ;
#11120=DIRECTION ( 'NONE',  ( -1.000000000000000000, -0.000000000000000000, -0.000000000000000000 ) ) ;
#11128=EDGE_LOOP ( 'NONE', ( #6307, #2487 ) ) ;
#11134=LINE ( 'NONE', #2161, #8006 ) ;
#11138=FACE_BOUND ( 'NONE', #1868, .T. ) ;
#11145=VERTEX_POINT ( 'NONE', #10046 ) ;
#11162=DIRECTION ( 'NONE',  ( -1.000000000000000000, -0.000000000000000000, -0.000000000000000000 ) ) ;
#11176=EDGE_CURVE ( 'NONE', #7332, #6004, #7419, .T. ) ;
#11177=LINE ( 'NONE', #5876, #4095 ) ;
#11182=CIRCLE ( 'NONE', #9850, 1.500000000000001332 ) ;
#11183=EDGE_LOOP ( 'NONE', ( #11236, #1792, #950, #8271 ) ) ;
#11185=ORIENTED_EDGE ( 'NONE', *, *, #11054, .F. ) ;
#11192=CARTESIAN_POINT ( 'NONE',  ( -80.00000000000002842, 38.02943725152282184, -1.499996628082202133 ) ) ;
#11195=CIRCLE ( 'NONE', #302, 1.500000000000001332 ) ;
#11196=EDGE_CURVE ( 'NONE', #1807, #9492, #320, .T. ) ;
#11200=CARTESIAN_POINT ( 'NONE',  ( -78.00000000000001421, 59.24264068711927678, 4.242644059037073312 ) ) ;
#11203=DIRECTION ( 'NONE',  ( -1.000000000000000000, -0.000000000000000000, -0.000000000000000000 ) ) ;
#11206=DIRECTION ( 'NONE',  ( -1.000000000000000000, -0.000000000000000000, -0.000000000000000000 ) ) ;
#11209=ORIENTED_EDGE ( 'NONE', *, *, #5055, .F. ) ;
#11212=PRODUCT_DEFINITION_SHAPE ( 'NONE', 'NONE',  #1895 ) ;
#11217=LINE ( 'NONE', #3027, #2415 ) ;
#11219=CYLINDRICAL_SURFACE ( 'NONE', #7231, 1.500000000000000000 ) ;
#11226=DIRECTION ( 'NONE',  ( -1.000000000000000000, -0.000000000000000000, -0.000000000000000000 ) ) ;
#11228=CARTESIAN_POINT ( 'NONE',  ( -78.00000000000000000, 54.99999999999999289, 3.371917797062584654E-06 ) ) ;
#11230=VERTEX_POINT ( 'NONE', #10171 ) ;
#11236=ORIENTED_EDGE ( 'NONE', *, *, #1030, .F. ) ;
#11240=CARTESIAN_POINT ( 'NONE',  ( -78.00000000000001421, 67.72792206135787296, 12.72792543327562775 ) ) ;
#11244=ORIENTED_EDGE ( 'NONE', *, *, #2183, .T. ) ;
#11246=FACE_BOUND ( 'NONE', #7291, .T. ) ;
#11249=EDGE_CURVE ( 'NONE', #4880, #9906, #7044, .T. ) ;
#11250=DIRECTION ( 'NONE',  ( 0.000000000000000000, 1.000000000000000000, 0.000000000000000000 ) ) ;
#11260=ORIENTED_EDGE ( 'NONE', *, *, #10177, .F. ) ;
#11263=DIRECTION ( 'NONE',  ( 0.000000000000000000, 1.000000000000000000, 0.000000000000000000 ) ) ;
#11264=CARTESIAN_POINT ( 'NONE',  ( -78.00000000000002842, 59.24264068711927678, 12.72792543327563131 ) ) ;
#11266=ORIENTED_EDGE ( 'NONE', *, *, #206, .F. ) ;
#11269=EDGE_LOOP ( 'NONE', ( #7258, #1920 ) ) ;
#11272=EDGE_CURVE ( 'NONE', #8769, #2643, #7607, .T. ) ;
#11280=EDGE_CURVE ( 'NONE', #932, #4386, #118, .T. ) ;
#11284=EDGE_LOOP ( 'NONE', ( #3796, #3729, #575, #8095 ) ) ;
#11297=AXIS2_PLACEMENT_3D ( 'NONE', #2587, #10656, #11496 ) ;
#11298=AXIS2_PLACEMENT_3D ( 'NONE', #8940, #7037, #6135 ) ;
#11299=DIRECTION ( 'NONE',  ( -1.000000000000000000, -0.000000000000000000, -0.000000000000000000 ) ) ;
#11326=CYLINDRICAL_SURFACE ( 'NONE', #8162, 1.499999999999999556 ) ;
#11327=ORIENTED_EDGE ( 'NONE', *, *, #9813, .T. ) ;
#11330=EDGE_LOOP ( 'NONE', ( #469, #4971 ) ) ;
#11337=VERTEX_POINT ( 'NONE', #10292 ) ;
#11338=DIRECTION ( 'NONE',  ( -1.000000000000000000, -0.000000000000000000, -0.000000000000000000 ) ) ;
#11354=CARTESIAN_POINT ( 'NONE',  ( -78.00000000000001421, 59.24264068711928388, -14.22791868944003646 ) ) ;
#11357=EDGE_CURVE ( 'NONE', #1492, #2813, #4011, .T. ) ;
#11362=CARTESIAN_POINT ( 'NONE',  ( -80.00000000000001421, 67.72792206135787296, -12.72791868944004534 ) ) ;
#11366=ORIENTED_EDGE ( 'NONE', *, *, #6504, .F. ) ;
#11369=DIRECTION ( 'NONE',  ( -1.000000000000000000, -0.000000000000000000, -0.000000000000000000 ) ) ;
#11370=CARTESIAN_POINT ( 'NONE',  ( -78.00000000000001421, 67.72792206135787296, 11.22792543327562775 ) ) ;
#11376=DIRECTION ( 'NONE',  ( -1.000000000000000000, -0.000000000000000000, -0.000000000000000000 ) ) ;
#11381=CARTESIAN_POINT ( 'NONE',  ( -80.00000000000002842, 54.99999999999998579, 9.985284746156354529 ) ) ;
#11390=ORIENTED_EDGE ( 'NONE', *, *, #7782, .T. ) ;
#11422=FACE_BOUND ( 'NONE', #8553, .T. ) ;
#11431=VECTOR ( 'NONE', #1964, 1000.000000000000000 ) ;
#11433=DIRECTION ( 'NONE',  ( -1.000000000000000000, -0.000000000000000000, -0.000000000000000000 ) ) ;
#11437=ORIENTED_EDGE ( 'NONE', *, *, #7825, .F. ) ;
#11441=EDGE_LOOP ( 'NONE', ( #5568, #4758 ) ) ;
#11444=ORIENTED_EDGE ( 'NONE', *, *, #10549, .F. ) ;
#11446=DIRECTION ( 'NONE',  ( 0.000000000000000000, 0.000000000000000000, 1.000000000000000000 ) ) ;
#11447=CARTESIAN_POINT ( 'NONE',  ( -78.00000000000000000, 54.99999999999999289, 3.371917797062584654E-06 ) ) ;
#11451=AXIS2_PLACEMENT_3D ( 'NONE', #9751, #4432, #4372 ) ;
#11454=DIRECTION ( 'NONE',  ( 0.000000000000000000, 1.000000000000000000, 0.000000000000000000 ) ) ;
#11463=ORIENTED_EDGE ( 'NONE', *, *, #3751, .F. ) ;
#11467=DIRECTION ( 'NONE',  ( -1.000000000000000000, -0.000000000000000000, -0.000000000000000000 ) ) ;
#11469=ORIENTED_EDGE ( 'NONE', *, *, #4890, .T. ) ;
#11473=CYLINDRICAL_SURFACE ( 'NONE', #9070, 1.500000000000000000 ) ;
#11480=FACE_BOUND ( 'NONE', #9383, .T. ) ;
#11481=VERTEX_POINT ( 'NONE', #7707 ) ;
#11487=ADVANCED_FACE ( 'NONE', ( #9370 ), #11219, .F. ) ;
#11489=DIRECTION ( 'NONE',  ( -1.000000000000000000, -0.000000000000000000, -0.000000000000000000 ) ) ;
#11496=DIRECTION ( 'NONE',  ( 0.000000000000000000, 0.000000000000000000, 1.000000000000000000 ) ) ;
#11497=CLOSED_SHELL ( 'NONE', ( #6966, #7106, #9280, #8592, #7195, #512, #4419, #3040, #11574, #4833, #2424, #1698, #11487, #6395, #8853, #6571, #803, #10176, #5080, #3795, #8580, #4676, #9450, #2857, #5015, #7314, #5140, #8288, #6028, #10683, #10247, #5432, #61, #263, #8330, #7507, #6001, #5426, #6470, #7935, #10910, #1592, #5745, #6440, #2734, #5528, #7421, #5545, #660, #11499, #10156, #9127, #6979, #10462, #957, #10400, #11562, #2397, #6224, #1914, #785, #5508 ) ) ;
#11499=ADVANCED_FACE ( 'NONE', ( #4832 ), #7589, .F. ) ;
#11504=VECTOR ( 'NONE', #11692, 1000.000000000000000 ) ;
#11517=EDGE_CURVE ( 'NONE', #9873, #43, #2042, .T. ) ;
#11526=VERTEX_POINT ( 'NONE', #8664 ) ;
#11528=CARTESIAN_POINT ( 'NONE',  ( -80.00000000000001421, 63.48528137423857487, -1.499996628082204797 ) ) ;
#11533=DIRECTION ( 'NONE',  ( -1.000000000000000000, -0.000000000000000000, -0.000000000000000000 ) ) ;
#11538=ORIENTED_EDGE ( 'NONE', *, *, #3317, .F. ) ;
#11540=CYLINDRICAL_SURFACE ( 'NONE', #7084, 1.499999999999999556 ) ;
#11541=PLANE ( 'NONE',  #3282 ) ;
#11552=DIRECTION ( 'NONE',  ( 0.000000000000000000, 0.000000000000000000, -1.000000000000000000 ) ) ;
#11556=VERTEX_POINT ( 'NONE', #6035 ) ;
#11562=ADVANCED_FACE ( 'NONE', ( #9556 ), #6934, .F. ) ;
#11568=EDGE_CURVE ( 'NONE', #3028, #4578, #3203, .T. ) ;
#11569=CIRCLE ( 'NONE', #7576, 1.500000000000001332 ) ;
#11570=CARTESIAN_POINT ( 'NONE',  ( -80.00000000000001421, 50.75735931288069480, -14.22791868944003646 ) ) ;
#11574=ADVANCED_FACE ( 'NONE', ( #676 ), #7761, .F. ) ;
#11575=ORIENTED_EDGE ( 'NONE', *, *, #1685, .T. ) ;
#11582=CIRCLE ( 'NONE', #7208, 1.500000000000001332 ) ;
#11586=CARTESIAN_POINT ( 'NONE',  ( -80.00000000000001421, 71.97056274847716395, 3.371917795327861178E-06 ) ) ;
#11592=AXIS2_PLACEMENT_3D ( 'NONE', #8442, #7367, #3886 ) ;
#11598=EDGE_LOOP ( 'NONE', ( #5312, #6196, #8342, #9005 ) ) ;
#11601=CARTESIAN_POINT ( 'NONE',  ( -80.00000000000001421, 67.72792206135787296, -5.742637315201482906 ) ) ;
#11603=CIRCLE ( 'NONE', #3013, 1.500000000000001332 ) ;
#11604=VERTEX_POINT ( 'NONE', #5248 ) ;
#11612=AXIS2_PLACEMENT_3D ( 'NONE', #5666, #11801, #9888 ) ;
#11614=FACE_OUTER_BOUND ( 'NONE', #11598, .T. ) ;
#11615=MECHANICAL_DESIGN_GEOMETRIC_PRESENTATION_REPRESENTATION('',(#3589),#1674);
#11617=CARTESIAN_POINT ( 'NONE',  ( -78.00000000000001421, 63.48528137423857487, 1.500003371917795425 ) ) ;
#11623=VECTOR ( 'NONE', #10419, 1000.000000000000000 ) ;
#11625=DIRECTION ( 'NONE',  ( -1.000000000000000000, -0.000000000000000000, -0.000000000000000000 ) ) ;
#11632=ORIENTED_EDGE ( 'NONE', *, *, #960, .F. ) ;
#11634=EDGE_CURVE ( 'NONE', #6038, #518, #5706, .T. ) ;
#11646=EDGE_CURVE ( 'NONE', #1618, #9349, #6813, .T. ) ;
#11649=DIRECTION ( 'NONE',  ( -1.000000000000000000, -0.000000000000000000, -0.000000000000000000 ) ) ;
#11654=VERTEX_POINT ( 'NONE', #5188 ) ;
#11660=EDGE_LOOP ( 'NONE', ( #8797, #7287, #8902, #2923 ) ) ;
#11668=CARTESIAN_POINT ( 'NONE',  ( -78.00000000000002842, 42.27207793864211283, 2.742644059037075976 ) ) ;
#11675=ORIENTED_EDGE ( 'NONE', *, *, #9295, .T. ) ;
#11684=CARTESIAN_POINT ( 'NONE',  ( -78.00000000000001421, 54.99999999999998579, -6.985278002320760571 ) ) ;
#11690=DIRECTION ( 'NONE',  ( -1.000000000000000000, -0.000000000000000000, -0.000000000000000000 ) ) ;
#11692=DIRECTION ( 'NONE',  ( -1.000000000000000000, -0.000000000000000000, -0.000000000000000000 ) ) ;
#11699=VECTOR ( 'NONE', #5181, 1000.000000000000000 ) ;
#11700=DIRECTION ( 'NONE',  ( -1.000000000000000000, -0.000000000000000000, -0.000000000000000000 ) ) ;
#11702=CARTESIAN_POINT ( 'NONE',  ( -80.00000000000002842, 42.27207793864211283, 12.72792543327562775 ) ) ;
#11718=EDGE_CURVE ( 'NONE', #8495, #1970, #3781, .T. ) ;
#11719=CARTESIAN_POINT ( 'NONE',  ( -80.00000000000002842, 46.51471862576140381, 6.985284746156355418 ) ) ;
#11720=DIRECTION ( 'NONE',  ( 0.000000000000000000, 0.000000000000000000, 1.000000000000000000 ) ) ;
#11731=ORIENTED_EDGE ( 'NONE', *, *, #6841, .F. ) ;
#11732=CARTESIAN_POINT ( 'NONE',  ( -78.00000000000001421, 59.24264068711927678, 2.742644059037073312 ) ) ;
#11743=LINE ( 'NONE', #5290, #8570 ) ;
#11759=VECTOR ( 'NONE', #10394, 1000.000000000000000 ) ;
#11773=ORIENTED_EDGE ( 'NONE', *, *, #1915, .F. ) ;
#11775=CYLINDRICAL_SURFACE ( 'NONE', #1328, 1.499999999999999556 ) ;
#11776=FACE_BOUND ( 'NONE', #2606, .T. ) ;
#11777=AXIS2_PLACEMENT_3D ( 'NONE', #3321, #6988, #10611 ) ;
#11779=VERTEX_POINT ( 'NONE', #10737 ) ;
#11785=EDGE_CURVE ( 'NONE', #1312, #849, #4938, .T. ) ;
#11786=CARTESIAN_POINT ( 'NONE',  ( -78.00000000000002842, 42.27207793864211283, 14.22792543327562775 ) ) ;
#11793=CIRCLE ( 'NONE', #11592, 1.500000000000001332 ) ;
#11797=AXIS2_PLACEMENT_3D ( 'NONE', #8448, #11063, #1065 ) ;
#11801=DIRECTION ( 'NONE',  ( -1.000000000000000000, -0.000000000000000000, -0.000000000000000000 ) ) ;
#11807=DIRECTION ( 'NONE',  ( -1.000000000000000000, -0.000000000000000000, -0.000000000000000000 ) ) ;
#11835=VECTOR ( 'NONE', #9146, 1000.000000000000000 ) ;
#11837=CIRCLE ( 'NONE', #10113, 1.500000000000001332 ) ;
#11843=DIRECTION ( 'NONE',  ( -1.000000000000000000, -0.000000000000000000, -0.000000000000000000 ) ) ;
#11845=AXIS2_PLACEMENT_3D ( 'NONE', #8466, #3850, #2951 ) ;
#11846=ORIENTED_EDGE ( 'NONE', *, *, #8290, .F. ) ;
#11853=EDGE_CURVE ( 'NONE', #1798, #10795, #7429, .T. ) ;
#11896=COLOUR_RGB('Off White',0.89,0.88,0.83);
#11897=FILL_AREA_STYLE_COLOUR('',#11896);
#11898=FILL_AREA_STYLE('',(#11897));
#11899=SURFACE_STYLE_FILL_AREA(#11898);
#11900=SURFACE_SIDE_STYLE('',(#11899));
#11901=SURFACE_STYLE_USAGE(.BOTH.,#11900);
#11902=PRESENTATION_STYLE_ASSIGNMENT((#11901));
ENDSEC;
END-ISO-10303-21;
